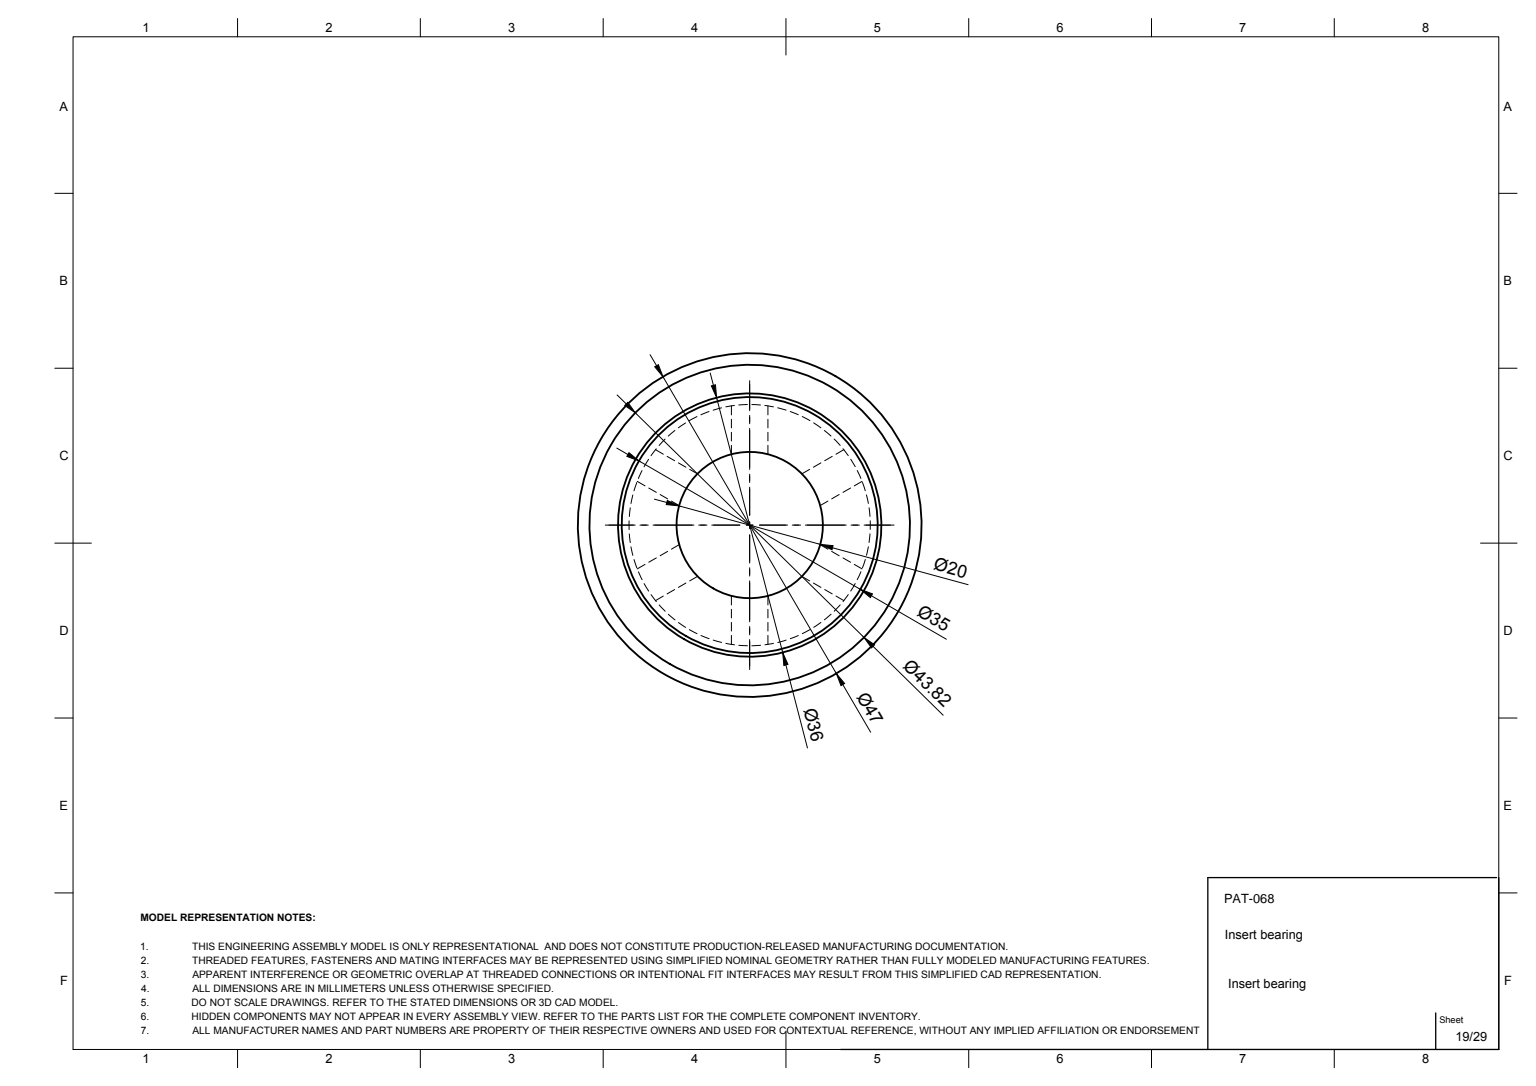
ISO-10303-21;
HEADER;
/* Generated by software containing ST-Developer
 * from STEP Tools, Inc. (www.steptools.com) 
 */

FILE_DESCRIPTION(
/* description */ ('Line shaft on three pillow blocks'),
/* implementation_level */ '2;1');

FILE_NAME(
/* name */ 'Insert bearing.step',
/* time_stamp */ '2026-10-27T10:49:19-07:00',
/* author */ (''),
/* organization */ (''),
/* preprocessor_version */ 'ST-DEVELOPER v20.2',
/* originating_system */ 'Autodesk Translation Framework v15.17.0.0',
/* authorisation */ '');

FILE_SCHEMA (('AUTOMOTIVE_DESIGN { 1 0 10303 214 3 1 1 }'));
ENDSEC;

DATA;
#10=MECHANICAL_DESIGN_GEOMETRIC_PRESENTATION_REPRESENTATION('',(#352,#353),#8377);
#223=B_SPLINE_CURVE_WITH_KNOTS('',3,(#7015,#7016,#7017,#7018,#7019,#7020,
#7021,#7022,#7023,#7024),.UNSPECIFIED.,.F.,.F.,(4,2,2,2,4),(1.13193471301885,
1.22626174930539,1.32058878559194,1.41491753480854,1.50924628402513),
 .UNSPECIFIED.);
#224=B_SPLINE_CURVE_WITH_KNOTS('',3,(#7026,#7027,#7028,#7029,#7030,#7031,
#7032,#7033,#7034,#7035,#7036,#7037,#7038,#7039,#7040,#7041,#7042,#7043),
 .UNSPECIFIED.,.F.,.F.,(4,2,2,2,2,2,2,2,4),(0.377311571006283,0.471638607292829,
0.565965643579376,0.66029439279597,0.754623142012565,0.84895189122916,0.943280640445754,
1.0376076767323,1.13193471301885),.UNSPECIFIED.);
#225=B_SPLINE_CURVE_WITH_KNOTS('',3,(#7044,#7045,#7046,#7047,#7048,#7049,
#7050,#7051,#7052,#7053),.UNSPECIFIED.,.F.,.F.,(4,2,2,2,4),(1.50924628402513,
1.60357503324173,1.69790378245832,1.79223081874487,1.88655785503141),
 .UNSPECIFIED.);
#226=B_SPLINE_CURVE_WITH_KNOTS('',3,(#7056,#7057,#7058,#7059,#7060,#7061,
#7062,#7063,#7064,#7065,#7066,#7067,#7068,#7069,#7070,#7071,#7072,#7073,
#7074,#7075,#7076,#7077,#7078,#7079,#7080,#7081,#7082,#7083,#7084,#7085,
#7086,#7087,#7088,#7089),.UNSPECIFIED.,.T.,.F.,(4,2,2,2,2,2,2,2,2,2,2,2,
2,2,2,2,4),(0.,0.0946120580087934,0.189224116017587,0.283822945575014,0.378421775132442,
0.47302060468987,0.567619434247297,0.662231492256091,0.756843550264884,
0.851455608273677,0.94606766628247,1.0406664958399,1.13526532539733,1.22986415495475,
1.32446298451218,1.41907504252097,1.51368710052977),.UNSPECIFIED.);
#227=B_SPLINE_CURVE_WITH_KNOTS('',3,(#7092,#7093,#7094,#7095,#7096,#7097,
#7098,#7099,#7100,#7101,#7102,#7103,#7104,#7105,#7106,#7107,#7108,#7109,
#7110,#7111,#7112,#7113,#7114,#7115,#7116,#7117,#7118,#7119,#7120,#7121,
#7122,#7123,#7124,#7125),.UNSPECIFIED.,.T.,.F.,(4,2,2,2,2,2,2,2,2,2,2,2,
2,2,2,2,4),(0.,0.0946120580087934,0.189224116017587,0.283822945575014,0.378421775132442,
0.47302060468987,0.567619434247297,0.66223149225609,0.756843550264884,0.851455608273677,
0.94606766628247,1.0406664958399,1.13526532539733,1.22986415495475,1.32446298451218,
1.41907504252097,1.51368710052977),.UNSPECIFIED.);
#228=B_SPLINE_CURVE_WITH_KNOTS('',3,(#7129,#7130,#7131,#7132,#7133,#7134,
#7135,#7136,#7137,#7138),.UNSPECIFIED.,.F.,.F.,(4,2,2,2,4),(1.13193471301885,
1.22626174930539,1.32058878559194,1.41491753480854,1.50924628402513),
 .UNSPECIFIED.);
#229=B_SPLINE_CURVE_WITH_KNOTS('',3,(#7140,#7141,#7142,#7143,#7144,#7145,
#7146,#7147,#7148,#7149,#7150,#7151,#7152,#7153,#7154,#7155,#7156,#7157),
 .UNSPECIFIED.,.F.,.F.,(4,2,2,2,2,2,2,2,4),(0.377311571006283,0.47163860729283,
0.565965643579376,0.660294392795971,0.754623142012565,0.84895189122916,
0.943280640445755,1.0376076767323,1.13193471301885),.UNSPECIFIED.);
#230=B_SPLINE_CURVE_WITH_KNOTS('',3,(#7158,#7159,#7160,#7161,#7162,#7163,
#7164,#7165,#7166,#7167),.UNSPECIFIED.,.F.,.F.,(4,2,2,2,4),(1.50924628402513,
1.60357503324173,1.69790378245832,1.79223081874487,1.88655785503141),
 .UNSPECIFIED.);
#231=B_SPLINE_CURVE_WITH_KNOTS('',3,(#7176,#7177,#7178,#7179,#7180,#7181,
#7182,#7183,#7184,#7185,#7186,#7187,#7188,#7189,#7190,#7191,#7192,#7193),
 .UNSPECIFIED.,.F.,.F.,(4,2,2,2,2,2,2,2,4),(0.377311571006282,0.471638607292829,
0.565965643579376,0.660294392795971,0.754623142012565,0.84895189122916,
0.943280640445754,1.0376076767323,1.13193471301885),.UNSPECIFIED.);
#232=B_SPLINE_CURVE_WITH_KNOTS('',3,(#7195,#7196,#7197,#7198,#7199,#7200,
#7201,#7202,#7203,#7204),.UNSPECIFIED.,.F.,.F.,(4,2,2,2,4),(1.13193471301885,
1.22626174930539,1.32058878559194,1.41491753480854,1.50924628402513),
 .UNSPECIFIED.);
#233=B_SPLINE_CURVE_WITH_KNOTS('',3,(#7205,#7206,#7207,#7208,#7209,#7210,
#7211,#7212,#7213,#7214),.UNSPECIFIED.,.F.,.F.,(4,2,2,2,4),(1.50924628402513,
1.60357503324172,1.69790378245832,1.79223081874487,1.88655785503141),
 .UNSPECIFIED.);
#234=B_SPLINE_CURVE_WITH_KNOTS('',3,(#7217,#7218,#7219,#7220,#7221,#7222,
#7223,#7224,#7225,#7226,#7227,#7228,#7229,#7230,#7231,#7232,#7233,#7234),
 .UNSPECIFIED.,.F.,.F.,(4,2,2,2,2,2,2,2,4),(0.377311571006283,0.47163860729283,
0.565965643579376,0.660294392795971,0.754623142012565,0.84895189122916,
0.943280640445754,1.0376076767323,1.13193471301885),.UNSPECIFIED.);
#235=B_SPLINE_CURVE_WITH_KNOTS('',3,(#7236,#7237,#7238,#7239,#7240,#7241,
#7242,#7243,#7244,#7245),.UNSPECIFIED.,.F.,.F.,(4,2,2,2,4),(1.13193471301885,
1.22626174930539,1.32058878559194,1.41491753480854,1.50924628402513),
 .UNSPECIFIED.);
#236=B_SPLINE_CURVE_WITH_KNOTS('',3,(#7246,#7247,#7248,#7249,#7250,#7251,
#7252,#7253,#7254,#7255),.UNSPECIFIED.,.F.,.F.,(4,2,2,2,4),(1.50924628402513,
1.60357503324173,1.69790378245832,1.79223081874487,1.88655785503141),
 .UNSPECIFIED.);
#237=B_SPLINE_CURVE_WITH_KNOTS('',3,(#7258,#7259,#7260,#7261,#7262,#7263,
#7264,#7265,#7266,#7267,#7268,#7269,#7270,#7271,#7272,#7273,#7274,#7275),
 .UNSPECIFIED.,.F.,.F.,(4,2,2,2,2,2,2,2,4),(0.377311571006282,0.471638607292829,
0.565965643579376,0.66029439279597,0.754623142012565,0.84895189122916,0.943280640445754,
1.0376076767323,1.13193471301885),.UNSPECIFIED.);
#238=B_SPLINE_CURVE_WITH_KNOTS('',3,(#7277,#7278,#7279,#7280,#7281,#7282,
#7283,#7284,#7285,#7286),.UNSPECIFIED.,.F.,.F.,(4,2,2,2,4),(1.13193471301885,
1.22626174930539,1.32058878559194,1.41491753480854,1.50924628402513),
 .UNSPECIFIED.);
#239=B_SPLINE_CURVE_WITH_KNOTS('',3,(#7287,#7288,#7289,#7290,#7291,#7292,
#7293,#7294,#7295,#7296),.UNSPECIFIED.,.F.,.F.,(4,2,2,2,4),(1.50924628402513,
1.60357503324172,1.69790378245832,1.79223081874487,1.88655785503141),
 .UNSPECIFIED.);
#240=B_SPLINE_CURVE_WITH_KNOTS('',3,(#7299,#7300,#7301,#7302,#7303,#7304,
#7305,#7306,#7307,#7308,#7309,#7310,#7311,#7312,#7313,#7314,#7315,#7316),
 .UNSPECIFIED.,.F.,.F.,(4,2,2,2,2,2,2,2,4),(0.377311571006283,0.471638607292829,
0.565965643579376,0.660294392795971,0.754623142012565,0.84895189122916,
0.943280640445755,1.0376076767323,1.13193471301885),.UNSPECIFIED.);
#241=B_SPLINE_CURVE_WITH_KNOTS('',3,(#7318,#7319,#7320,#7321,#7322,#7323,
#7324,#7325,#7326,#7327),.UNSPECIFIED.,.F.,.F.,(4,2,2,2,4),(1.13193471301885,
1.22626174930539,1.32058878559194,1.41491753480854,1.50924628402513),
 .UNSPECIFIED.);
#242=B_SPLINE_CURVE_WITH_KNOTS('',3,(#7328,#7329,#7330,#7331,#7332,#7333,
#7334,#7335,#7336,#7337),.UNSPECIFIED.,.F.,.F.,(4,2,2,2,4),(1.50924628402513,
1.60357503324172,1.69790378245832,1.79223081874487,1.88655785503141),
 .UNSPECIFIED.);
#243=B_SPLINE_CURVE_WITH_KNOTS('',3,(#7341,#7342,#7343,#7344,#7345,#7346,
#7347,#7348,#7349,#7350,#7351,#7352,#7353,#7354,#7355,#7356,#7357,#7358,
#7359,#7360,#7361,#7362,#7363,#7364,#7365,#7366,#7367,#7368,#7369,#7370,
#7371,#7372,#7373,#7374),.UNSPECIFIED.,.T.,.F.,(4,2,2,2,2,2,2,2,2,2,2,2,
2,2,2,2,4),(0.,0.0946120580087934,0.189224116017587,0.283822945575014,0.378421775132442,
0.47302060468987,0.567619434247297,0.66223149225609,0.756843550264884,0.851455608273677,
0.94606766628247,1.0406664958399,1.13526532539733,1.22986415495475,1.32446298451218,
1.41907504252097,1.51368710052977),.UNSPECIFIED.);
#244=B_SPLINE_CURVE_WITH_KNOTS('',3,(#7377,#7378,#7379,#7380,#7381,#7382,
#7383,#7384,#7385,#7386,#7387,#7388,#7389,#7390,#7391,#7392,#7393,#7394,
#7395,#7396,#7397,#7398,#7399,#7400,#7401,#7402,#7403,#7404,#7405,#7406,
#7407,#7408,#7409,#7410),.UNSPECIFIED.,.T.,.F.,(4,2,2,2,2,2,2,2,2,2,2,2,
2,2,2,2,4),(0.,0.0946120580087934,0.189224116017587,0.283822945575014,0.378421775132442,
0.47302060468987,0.567619434247297,0.66223149225609,0.756843550264884,0.851455608273677,
0.94606766628247,1.0406664958399,1.13526532539733,1.22986415495475,1.32446298451218,
1.41907504252097,1.51368710052977),.UNSPECIFIED.);
#245=B_SPLINE_CURVE_WITH_KNOTS('',3,(#7415,#7416,#7417,#7418,#7419,#7420,
#7421,#7422,#7423,#7424,#7425,#7426,#7427,#7428,#7429,#7430,#7431,#7432,
#7433,#7434,#7435,#7436,#7437,#7438,#7439,#7440,#7441,#7442,#7443,#7444,
#7445,#7446,#7447,#7448),.UNSPECIFIED.,.T.,.F.,(4,2,2,2,2,2,2,2,2,2,2,2,
2,2,2,2,4),(0.,0.0946120580087934,0.189224116017587,0.283822945575014,0.378421775132442,
0.47302060468987,0.567619434247297,0.66223149225609,0.756843550264884,0.851455608273677,
0.94606766628247,1.0406664958399,1.13526532539733,1.22986415495475,1.32446298451218,
1.41907504252097,1.51368710052977),.UNSPECIFIED.);
#246=B_SPLINE_CURVE_WITH_KNOTS('',3,(#7451,#7452,#7453,#7454,#7455,#7456,
#7457,#7458,#7459,#7460,#7461,#7462,#7463,#7464,#7465,#7466,#7467,#7468,
#7469,#7470,#7471,#7472,#7473,#7474,#7475,#7476,#7477,#7478,#7479,#7480,
#7481,#7482,#7483,#7484),.UNSPECIFIED.,.T.,.F.,(4,2,2,2,2,2,2,2,2,2,2,2,
2,2,2,2,4),(0.,0.0946120580087934,0.189224116017587,0.283822945575014,0.378421775132442,
0.47302060468987,0.567619434247297,0.66223149225609,0.756843550264884,0.851455608273677,
0.94606766628247,1.0406664958399,1.13526532539733,1.22986415495475,1.32446298451218,
1.41907504252097,1.51368710052977),.UNSPECIFIED.);
#264=SPHERICAL_SURFACE('',#4873,2.35);
#298=SHAPE_REPRESENTATION_RELATIONSHIP('SRR','None',#8514,#325);
#325=ADVANCED_BREP_SHAPE_REPRESENTATION('',(#379,#380),#8363);
#352=STYLED_ITEM('',(#8718),#379);
#353=STYLED_ITEM('',(#8718),#380);
#379=MANIFOLD_SOLID_BREP('Body1',#4339);
#380=MANIFOLD_SOLID_BREP('Body2',#4340);
#440=FACE_BOUND('',#1075,.T.);
#441=FACE_BOUND('',#1077,.T.);
#442=FACE_BOUND('',#1078,.T.);
#443=FACE_BOUND('',#1080,.T.);
#444=FACE_BOUND('',#1084,.T.);
#445=FACE_BOUND('',#1085,.T.);
#446=FACE_BOUND('',#1086,.T.);
#447=FACE_BOUND('',#1087,.T.);
#448=FACE_BOUND('',#1088,.T.);
#449=FACE_BOUND('',#1089,.T.);
#450=FACE_BOUND('',#1095,.T.);
#451=FACE_BOUND('',#1097,.T.);
#452=FACE_BOUND('',#1100,.T.);
#453=FACE_BOUND('',#1102,.T.);
#454=FACE_BOUND('',#1103,.T.);
#455=FACE_BOUND('',#1104,.T.);
#456=FACE_BOUND('',#1105,.T.);
#457=FACE_BOUND('',#1106,.T.);
#458=FACE_BOUND('',#1107,.T.);
#566=PLANE('',#4871);
#567=PLANE('',#4876);
#568=PLANE('',#4886);
#569=PLANE('',#4888);
#570=PLANE('',#4892);
#772=FACE_OUTER_BOUND('',#1073,.T.);
#773=FACE_OUTER_BOUND('',#1074,.T.);
#774=FACE_OUTER_BOUND('',#1076,.T.);
#775=FACE_OUTER_BOUND('',#1079,.T.);
#776=FACE_OUTER_BOUND('',#1081,.T.);
#777=FACE_OUTER_BOUND('',#1082,.T.);
#778=FACE_OUTER_BOUND('',#1083,.T.);
#779=FACE_OUTER_BOUND('',#1090,.T.);
#780=FACE_OUTER_BOUND('',#1091,.T.);
#781=FACE_OUTER_BOUND('',#1092,.T.);
#782=FACE_OUTER_BOUND('',#1093,.T.);
#783=FACE_OUTER_BOUND('',#1094,.T.);
#784=FACE_OUTER_BOUND('',#1096,.T.);
#785=FACE_OUTER_BOUND('',#1098,.T.);
#786=FACE_OUTER_BOUND('',#1099,.T.);
#787=FACE_OUTER_BOUND('',#1101,.T.);
#1073=EDGE_LOOP('',(#3423,#3424,#3425,#3426));
#1074=EDGE_LOOP('',(#3427));
#1075=EDGE_LOOP('',(#3428));
#1076=EDGE_LOOP('',(#3429,#3430));
#1077=EDGE_LOOP('',(#3431));
#1078=EDGE_LOOP('',(#3432));
#1079=EDGE_LOOP('',(#3433));
#1080=EDGE_LOOP('',(#3434));
#1081=EDGE_LOOP('',(#3435,#3436,#3437,#3438,#3439,#3440));
#1082=EDGE_LOOP('',(#3441,#3442,#3443,#3444,#3445,#3446));
#1083=EDGE_LOOP('',(#3447,#3448,#3449,#3450));
#1084=EDGE_LOOP('',(#3451,#3452,#3453));
#1085=EDGE_LOOP('',(#3454,#3455,#3456));
#1086=EDGE_LOOP('',(#3457,#3458,#3459));
#1087=EDGE_LOOP('',(#3460,#3461,#3462));
#1088=EDGE_LOOP('',(#3463,#3464,#3465));
#1089=EDGE_LOOP('',(#3466,#3467,#3468));
#1090=EDGE_LOOP('',(#3469,#3470,#3471,#3472,#3473,#3474));
#1091=EDGE_LOOP('',(#3475,#3476,#3477,#3478,#3479,#3480));
#1092=EDGE_LOOP('',(#3481,#3482,#3483,#3484,#3485,#3486));
#1093=EDGE_LOOP('',(#3487,#3488,#3489,#3490,#3491,#3492));
#1094=EDGE_LOOP('',(#3493));
#1095=EDGE_LOOP('',(#3494));
#1096=EDGE_LOOP('',(#3495));
#1097=EDGE_LOOP('',(#3496));
#1098=EDGE_LOOP('',(#3497,#3498,#3499,#3500));
#1099=EDGE_LOOP('',(#3501));
#1100=EDGE_LOOP('',(#3502));
#1101=EDGE_LOOP('',(#3503,#3504,#3505,#3506));
#1102=EDGE_LOOP('',(#3507));
#1103=EDGE_LOOP('',(#3508));
#1104=EDGE_LOOP('',(#3509));
#1105=EDGE_LOOP('',(#3510));
#1106=EDGE_LOOP('',(#3511));
#1107=EDGE_LOOP('',(#3512));
#1413=LINE('',#7000,#1740);
#1414=LINE('',#7055,#1741);
#1415=LINE('',#7127,#1742);
#1416=LINE('',#7172,#1743);
#1417=LINE('',#7340,#1744);
#1418=LINE('',#7411,#1745);
#1419=LINE('',#7414,#1746);
#1420=LINE('',#7485,#1747);
#1421=LINE('',#7495,#1748);
#1422=LINE('',#7500,#1749);
#1740=VECTOR('',#5740,1.8);
#1741=VECTOR('',#5757,0.25);
#1742=VECTOR('',#5760,0.25);
#1743=VECTOR('',#5765,1.65);
#1744=VECTOR('',#5770,0.25);
#1745=VECTOR('',#5773,0.25);
#1746=VECTOR('',#5776,0.25);
#1747=VECTOR('',#5779,0.25);
#1748=VECTOR('',#5792,1.75);
#1749=VECTOR('',#5799,1.);
#1988=CIRCLE('',#4869,1.8);
#1989=CIRCLE('',#4870,1.8);
#1990=CIRCLE('',#4872,2.19089023002066);
#1991=CIRCLE('',#4874,2.35);
#1992=CIRCLE('',#4875,2.19089023002066);
#1993=CIRCLE('',#4880,1.65);
#1994=CIRCLE('',#4881,1.65);
#1995=CIRCLE('',#4887,1.);
#1996=CIRCLE('',#4889,1.75);
#1997=CIRCLE('',#4891,1.75);
#1998=CIRCLE('',#4893,1.);
#2226=VERTEX_POINT('',#6997);
#2227=VERTEX_POINT('',#6999);
#2228=VERTEX_POINT('',#7003);
#2229=VERTEX_POINT('',#7006);
#2230=VERTEX_POINT('',#7007);
#2231=VERTEX_POINT('',#7009);
#2232=VERTEX_POINT('',#7013);
#2233=VERTEX_POINT('',#7014);
#2234=VERTEX_POINT('',#7025);
#2235=VERTEX_POINT('',#7054);
#2236=VERTEX_POINT('',#7091);
#2237=VERTEX_POINT('',#7126);
#2238=VERTEX_POINT('',#7128);
#2239=VERTEX_POINT('',#7139);
#2240=VERTEX_POINT('',#7169);
#2241=VERTEX_POINT('',#7171);
#2242=VERTEX_POINT('',#7174);
#2243=VERTEX_POINT('',#7175);
#2244=VERTEX_POINT('',#7194);
#2245=VERTEX_POINT('',#7215);
#2246=VERTEX_POINT('',#7216);
#2247=VERTEX_POINT('',#7235);
#2248=VERTEX_POINT('',#7256);
#2249=VERTEX_POINT('',#7257);
#2250=VERTEX_POINT('',#7276);
#2251=VERTEX_POINT('',#7297);
#2252=VERTEX_POINT('',#7298);
#2253=VERTEX_POINT('',#7317);
#2254=VERTEX_POINT('',#7339);
#2255=VERTEX_POINT('',#7376);
#2256=VERTEX_POINT('',#7413);
#2257=VERTEX_POINT('',#7450);
#2258=VERTEX_POINT('',#7487);
#2259=VERTEX_POINT('',#7490);
#2260=VERTEX_POINT('',#7493);
#2261=VERTEX_POINT('',#7497);
#2660=EDGE_CURVE('',#2226,#2226,#1988,.T.);
#2661=EDGE_CURVE('',#2226,#2227,#1413,.T.);
#2662=EDGE_CURVE('',#2227,#2227,#1989,.T.);
#2663=EDGE_CURVE('',#2228,#2228,#1990,.T.);
#2664=EDGE_CURVE('',#2229,#2230,#1991,.T.);
#2665=EDGE_CURVE('',#2231,#2231,#1992,.T.);
#2666=EDGE_CURVE('',#2232,#2233,#223,.T.);
#2667=EDGE_CURVE('',#2234,#2232,#224,.T.);
#2668=EDGE_CURVE('',#2233,#2234,#225,.T.);
#2669=EDGE_CURVE('',#2233,#2235,#1414,.T.);
#2670=EDGE_CURVE('',#2235,#2235,#226,.T.);
#2671=EDGE_CURVE('',#2236,#2236,#227,.T.);
#2672=EDGE_CURVE('',#2236,#2237,#1415,.T.);
#2673=EDGE_CURVE('',#2238,#2237,#228,.T.);
#2674=EDGE_CURVE('',#2239,#2238,#229,.T.);
#2675=EDGE_CURVE('',#2237,#2239,#230,.T.);
#2676=EDGE_CURVE('',#2240,#2240,#1993,.T.);
#2677=EDGE_CURVE('',#2240,#2241,#1416,.T.);
#2678=EDGE_CURVE('',#2241,#2241,#1994,.T.);
#2679=EDGE_CURVE('',#2242,#2243,#231,.T.);
#2680=EDGE_CURVE('',#2243,#2244,#232,.T.);
#2681=EDGE_CURVE('',#2244,#2242,#233,.T.);
#2682=EDGE_CURVE('',#2245,#2246,#234,.T.);
#2683=EDGE_CURVE('',#2246,#2247,#235,.T.);
#2684=EDGE_CURVE('',#2247,#2245,#236,.T.);
#2685=EDGE_CURVE('',#2248,#2249,#237,.T.);
#2686=EDGE_CURVE('',#2249,#2250,#238,.T.);
#2687=EDGE_CURVE('',#2250,#2248,#239,.T.);
#2688=EDGE_CURVE('',#2251,#2252,#240,.T.);
#2689=EDGE_CURVE('',#2252,#2253,#241,.T.);
#2690=EDGE_CURVE('',#2253,#2251,#242,.T.);
#2691=EDGE_CURVE('',#2244,#2254,#1417,.T.);
#2692=EDGE_CURVE('',#2254,#2254,#243,.T.);
#2693=EDGE_CURVE('',#2255,#2255,#244,.T.);
#2694=EDGE_CURVE('',#2255,#2247,#1418,.T.);
#2695=EDGE_CURVE('',#2250,#2256,#1419,.T.);
#2696=EDGE_CURVE('',#2256,#2256,#245,.T.);
#2697=EDGE_CURVE('',#2257,#2257,#246,.T.);
#2698=EDGE_CURVE('',#2257,#2253,#1420,.T.);
#2699=EDGE_CURVE('',#2258,#2258,#1995,.T.);
#2700=EDGE_CURVE('',#2259,#2259,#1996,.T.);
#2701=EDGE_CURVE('',#2260,#2260,#1997,.T.);
#2702=EDGE_CURVE('',#2260,#2259,#1421,.T.);
#2703=EDGE_CURVE('',#2261,#2261,#1998,.T.);
#2704=EDGE_CURVE('',#2261,#2258,#1422,.T.);
#3423=ORIENTED_EDGE('',*,*,#2660,.T.);
#3424=ORIENTED_EDGE('',*,*,#2661,.T.);
#3425=ORIENTED_EDGE('',*,*,#2662,.F.);
#3426=ORIENTED_EDGE('',*,*,#2661,.F.);
#3427=ORIENTED_EDGE('',*,*,#2663,.F.);
#3428=ORIENTED_EDGE('',*,*,#2662,.T.);
#3429=ORIENTED_EDGE('',*,*,#2664,.T.);
#3430=ORIENTED_EDGE('',*,*,#2664,.F.);
#3431=ORIENTED_EDGE('',*,*,#2663,.T.);
#3432=ORIENTED_EDGE('',*,*,#2665,.F.);
#3433=ORIENTED_EDGE('',*,*,#2665,.T.);
#3434=ORIENTED_EDGE('',*,*,#2660,.F.);
#3435=ORIENTED_EDGE('',*,*,#2666,.F.);
#3436=ORIENTED_EDGE('',*,*,#2667,.F.);
#3437=ORIENTED_EDGE('',*,*,#2668,.F.);
#3438=ORIENTED_EDGE('',*,*,#2669,.T.);
#3439=ORIENTED_EDGE('',*,*,#2670,.F.);
#3440=ORIENTED_EDGE('',*,*,#2669,.F.);
#3441=ORIENTED_EDGE('',*,*,#2671,.F.);
#3442=ORIENTED_EDGE('',*,*,#2672,.T.);
#3443=ORIENTED_EDGE('',*,*,#2673,.F.);
#3444=ORIENTED_EDGE('',*,*,#2674,.F.);
#3445=ORIENTED_EDGE('',*,*,#2675,.F.);
#3446=ORIENTED_EDGE('',*,*,#2672,.F.);
#3447=ORIENTED_EDGE('',*,*,#2676,.F.);
#3448=ORIENTED_EDGE('',*,*,#2677,.T.);
#3449=ORIENTED_EDGE('',*,*,#2678,.T.);
#3450=ORIENTED_EDGE('',*,*,#2677,.F.);
#3451=ORIENTED_EDGE('',*,*,#2667,.T.);
#3452=ORIENTED_EDGE('',*,*,#2666,.T.);
#3453=ORIENTED_EDGE('',*,*,#2668,.T.);
#3454=ORIENTED_EDGE('',*,*,#2674,.T.);
#3455=ORIENTED_EDGE('',*,*,#2673,.T.);
#3456=ORIENTED_EDGE('',*,*,#2675,.T.);
#3457=ORIENTED_EDGE('',*,*,#2679,.T.);
#3458=ORIENTED_EDGE('',*,*,#2680,.T.);
#3459=ORIENTED_EDGE('',*,*,#2681,.T.);
#3460=ORIENTED_EDGE('',*,*,#2682,.T.);
#3461=ORIENTED_EDGE('',*,*,#2683,.T.);
#3462=ORIENTED_EDGE('',*,*,#2684,.T.);
#3463=ORIENTED_EDGE('',*,*,#2685,.T.);
#3464=ORIENTED_EDGE('',*,*,#2686,.T.);
#3465=ORIENTED_EDGE('',*,*,#2687,.T.);
#3466=ORIENTED_EDGE('',*,*,#2688,.T.);
#3467=ORIENTED_EDGE('',*,*,#2689,.T.);
#3468=ORIENTED_EDGE('',*,*,#2690,.T.);
#3469=ORIENTED_EDGE('',*,*,#2680,.F.);
#3470=ORIENTED_EDGE('',*,*,#2679,.F.);
#3471=ORIENTED_EDGE('',*,*,#2681,.F.);
#3472=ORIENTED_EDGE('',*,*,#2691,.T.);
#3473=ORIENTED_EDGE('',*,*,#2692,.F.);
#3474=ORIENTED_EDGE('',*,*,#2691,.F.);
#3475=ORIENTED_EDGE('',*,*,#2693,.F.);
#3476=ORIENTED_EDGE('',*,*,#2694,.T.);
#3477=ORIENTED_EDGE('',*,*,#2683,.F.);
#3478=ORIENTED_EDGE('',*,*,#2682,.F.);
#3479=ORIENTED_EDGE('',*,*,#2684,.F.);
#3480=ORIENTED_EDGE('',*,*,#2694,.F.);
#3481=ORIENTED_EDGE('',*,*,#2686,.F.);
#3482=ORIENTED_EDGE('',*,*,#2685,.F.);
#3483=ORIENTED_EDGE('',*,*,#2687,.F.);
#3484=ORIENTED_EDGE('',*,*,#2695,.T.);
#3485=ORIENTED_EDGE('',*,*,#2696,.F.);
#3486=ORIENTED_EDGE('',*,*,#2695,.F.);
#3487=ORIENTED_EDGE('',*,*,#2697,.F.);
#3488=ORIENTED_EDGE('',*,*,#2698,.T.);
#3489=ORIENTED_EDGE('',*,*,#2689,.F.);
#3490=ORIENTED_EDGE('',*,*,#2688,.F.);
#3491=ORIENTED_EDGE('',*,*,#2690,.F.);
#3492=ORIENTED_EDGE('',*,*,#2698,.F.);
#3493=ORIENTED_EDGE('',*,*,#2678,.F.);
#3494=ORIENTED_EDGE('',*,*,#2699,.T.);
#3495=ORIENTED_EDGE('',*,*,#2700,.F.);
#3496=ORIENTED_EDGE('',*,*,#2676,.T.);
#3497=ORIENTED_EDGE('',*,*,#2701,.F.);
#3498=ORIENTED_EDGE('',*,*,#2702,.T.);
#3499=ORIENTED_EDGE('',*,*,#2700,.T.);
#3500=ORIENTED_EDGE('',*,*,#2702,.F.);
#3501=ORIENTED_EDGE('',*,*,#2701,.T.);
#3502=ORIENTED_EDGE('',*,*,#2703,.F.);
#3503=ORIENTED_EDGE('',*,*,#2703,.T.);
#3504=ORIENTED_EDGE('',*,*,#2704,.T.);
#3505=ORIENTED_EDGE('',*,*,#2699,.F.);
#3506=ORIENTED_EDGE('',*,*,#2704,.F.);
#3507=ORIENTED_EDGE('',*,*,#2671,.T.);
#3508=ORIENTED_EDGE('',*,*,#2670,.T.);
#3509=ORIENTED_EDGE('',*,*,#2693,.T.);
#3510=ORIENTED_EDGE('',*,*,#2692,.T.);
#3511=ORIENTED_EDGE('',*,*,#2697,.T.);
#3512=ORIENTED_EDGE('',*,*,#2696,.T.);
#4036=CYLINDRICAL_SURFACE('',#4868,1.8);
#4037=CYLINDRICAL_SURFACE('',#4877,0.25);
#4038=CYLINDRICAL_SURFACE('',#4878,0.25);
#4039=CYLINDRICAL_SURFACE('',#4879,1.65);
#4040=CYLINDRICAL_SURFACE('',#4882,0.25);
#4041=CYLINDRICAL_SURFACE('',#4883,0.25);
#4042=CYLINDRICAL_SURFACE('',#4884,0.25);
#4043=CYLINDRICAL_SURFACE('',#4885,0.25);
#4044=CYLINDRICAL_SURFACE('',#4890,1.75);
#4045=CYLINDRICAL_SURFACE('',#4894,1.);
#4190=ADVANCED_FACE('',(#772),#4036,.F.);
#4191=ADVANCED_FACE('',(#773,#440),#566,.T.);
#4192=ADVANCED_FACE('',(#774,#441,#442),#264,.T.);
#4193=ADVANCED_FACE('',(#775,#443),#567,.T.);
#4194=ADVANCED_FACE('',(#776),#4037,.F.);
#4195=ADVANCED_FACE('',(#777),#4038,.F.);
#4196=ADVANCED_FACE('',(#778,#444,#445,#446,#447,#448,#449),#4039,.T.);
#4197=ADVANCED_FACE('',(#779),#4040,.F.);
#4198=ADVANCED_FACE('',(#780),#4041,.F.);
#4199=ADVANCED_FACE('',(#781),#4042,.F.);
#4200=ADVANCED_FACE('',(#782),#4043,.F.);
#4201=ADVANCED_FACE('',(#783,#450),#568,.T.);
#4202=ADVANCED_FACE('',(#784,#451),#569,.T.);
#4203=ADVANCED_FACE('',(#785),#4044,.T.);
#4204=ADVANCED_FACE('',(#786,#452),#570,.T.);
#4205=ADVANCED_FACE('',(#787,#453,#454,#455,#456,#457,#458),#4045,.F.);
#4339=CLOSED_SHELL('',(#4190,#4191,#4192,#4193));
#4340=CLOSED_SHELL('',(#4194,#4195,#4196,#4197,#4198,#4199,#4200,#4201,
#4202,#4203,#4204,#4205));
#4867=AXIS2_PLACEMENT_3D('',#6995,#5734,#5735);
#4868=AXIS2_PLACEMENT_3D('',#6996,#5736,#5737);
#4869=AXIS2_PLACEMENT_3D('',#6998,#5738,#5739);
#4870=AXIS2_PLACEMENT_3D('',#7001,#5741,#5742);
#4871=AXIS2_PLACEMENT_3D('',#7002,#5743,#5744);
#4872=AXIS2_PLACEMENT_3D('',#7004,#5745,#5746);
#4873=AXIS2_PLACEMENT_3D('',#7005,#5747,#5748);
#4874=AXIS2_PLACEMENT_3D('',#7008,#5749,#5750);
#4875=AXIS2_PLACEMENT_3D('',#7010,#5751,#5752);
#4876=AXIS2_PLACEMENT_3D('',#7011,#5753,#5754);
#4877=AXIS2_PLACEMENT_3D('',#7012,#5755,#5756);
#4878=AXIS2_PLACEMENT_3D('',#7090,#5758,#5759);
#4879=AXIS2_PLACEMENT_3D('',#7168,#5761,#5762);
#4880=AXIS2_PLACEMENT_3D('',#7170,#5763,#5764);
#4881=AXIS2_PLACEMENT_3D('',#7173,#5766,#5767);
#4882=AXIS2_PLACEMENT_3D('',#7338,#5768,#5769);
#4883=AXIS2_PLACEMENT_3D('',#7375,#5771,#5772);
#4884=AXIS2_PLACEMENT_3D('',#7412,#5774,#5775);
#4885=AXIS2_PLACEMENT_3D('',#7449,#5777,#5778);
#4886=AXIS2_PLACEMENT_3D('',#7486,#5780,#5781);
#4887=AXIS2_PLACEMENT_3D('',#7488,#5782,#5783);
#4888=AXIS2_PLACEMENT_3D('',#7489,#5784,#5785);
#4889=AXIS2_PLACEMENT_3D('',#7491,#5786,#5787);
#4890=AXIS2_PLACEMENT_3D('',#7492,#5788,#5789);
#4891=AXIS2_PLACEMENT_3D('',#7494,#5790,#5791);
#4892=AXIS2_PLACEMENT_3D('',#7496,#5793,#5794);
#4893=AXIS2_PLACEMENT_3D('',#7498,#5795,#5796);
#4894=AXIS2_PLACEMENT_3D('',#7499,#5797,#5798);
#5734=DIRECTION('axis',(0.,0.,1.));
#5735=DIRECTION('refdir',(1.,0.,0.));
#5736=DIRECTION('center_axis',(0.,-1.,0.));
#5737=DIRECTION('ref_axis',(1.,0.,0.));
#5738=DIRECTION('center_axis',(0.,-1.,0.));
#5739=DIRECTION('ref_axis',(1.,0.,0.));
#5740=DIRECTION('',(0.,1.,0.));
#5741=DIRECTION('center_axis',(0.,-1.,0.));
#5742=DIRECTION('ref_axis',(1.,0.,0.));
#5743=DIRECTION('center_axis',(0.,1.,0.));
#5744=DIRECTION('ref_axis',(0.,0.,1.));
#5745=DIRECTION('center_axis',(0.,-1.,0.));
#5746=DIRECTION('ref_axis',(1.,0.,0.));
#5747=DIRECTION('center_axis',(6.12323399573677E-17,0.,1.));
#5748=DIRECTION('ref_axis',(1.,0.,0.));
#5749=DIRECTION('center_axis',(1.22464679914735E-16,-1.,0.));
#5750=DIRECTION('ref_axis',(-1.,-1.22464679914735E-16,0.));
#5751=DIRECTION('center_axis',(0.,-1.,0.));
#5752=DIRECTION('ref_axis',(1.,0.,0.));
#5753=DIRECTION('center_axis',(0.,-1.,0.));
#5754=DIRECTION('ref_axis',(0.,0.,-1.));
#5755=DIRECTION('center_axis',(-0.866025403784438,0.,-0.5));
#5756=DIRECTION('ref_axis',(-0.5,0.,0.866025403784438));
#5757=DIRECTION('',(-0.866025403784438,0.,-0.5));
#5758=DIRECTION('center_axis',(-0.866025403784438,0.,-0.5));
#5759=DIRECTION('ref_axis',(-0.5,0.,0.866025403784438));
#5760=DIRECTION('',(-0.866025403784438,0.,-0.5));
#5761=DIRECTION('center_axis',(0.,-1.,0.));
#5762=DIRECTION('ref_axis',(1.,0.,0.));
#5763=DIRECTION('center_axis',(0.,-1.,0.));
#5764=DIRECTION('ref_axis',(1.,0.,0.));
#5765=DIRECTION('',(0.,1.,0.));
#5766=DIRECTION('center_axis',(0.,-1.,0.));
#5767=DIRECTION('ref_axis',(1.,0.,0.));
#5768=DIRECTION('center_axis',(0.866025403784439,0.,-0.5));
#5769=DIRECTION('ref_axis',(-0.5,0.,-0.866025403784439));
#5770=DIRECTION('',(0.866025403784439,0.,-0.5));
#5771=DIRECTION('center_axis',(0.866025403784439,0.,-0.5));
#5772=DIRECTION('ref_axis',(-0.5,0.,-0.866025403784439));
#5773=DIRECTION('',(0.866025403784439,0.,-0.5));
#5774=DIRECTION('center_axis',(0.,0.,1.));
#5775=DIRECTION('ref_axis',(1.,0.,0.));
#5776=DIRECTION('',(0.,0.,1.));
#5777=DIRECTION('center_axis',(0.,0.,1.));
#5778=DIRECTION('ref_axis',(1.,0.,0.));
#5779=DIRECTION('',(0.,0.,1.));
#5780=DIRECTION('center_axis',(0.,1.,0.));
#5781=DIRECTION('ref_axis',(0.,0.,1.));
#5782=DIRECTION('center_axis',(0.,-1.,0.));
#5783=DIRECTION('ref_axis',(1.,0.,0.));
#5784=DIRECTION('center_axis',(0.,1.,0.));
#5785=DIRECTION('ref_axis',(0.,0.,1.));
#5786=DIRECTION('center_axis',(0.,-1.,0.));
#5787=DIRECTION('ref_axis',(1.,0.,0.));
#5788=DIRECTION('center_axis',(0.,-1.,0.));
#5789=DIRECTION('ref_axis',(1.,0.,0.));
#5790=DIRECTION('center_axis',(0.,-1.,0.));
#5791=DIRECTION('ref_axis',(1.,0.,0.));
#5792=DIRECTION('',(0.,1.,0.));
#5793=DIRECTION('center_axis',(0.,-1.,0.));
#5794=DIRECTION('ref_axis',(0.,0.,-1.));
#5795=DIRECTION('center_axis',(0.,-1.,0.));
#5796=DIRECTION('ref_axis',(1.,0.,0.));
#5797=DIRECTION('center_axis',(0.,-1.,0.));
#5798=DIRECTION('ref_axis',(1.,0.,0.));
#5799=DIRECTION('',(0.,1.,0.));
#6995=CARTESIAN_POINT('',(0.,0.,0.));
#6996=CARTESIAN_POINT('Origin',(0.,0.,0.));
#6997=CARTESIAN_POINT('',(-1.8,-0.85,-2.20436423846524E-16));
#6998=CARTESIAN_POINT('Origin',(0.,-0.85,0.));
#6999=CARTESIAN_POINT('',(-1.8,0.85,-2.20436423846524E-16));
#7000=CARTESIAN_POINT('',(-1.8,0.,-2.20436423846524E-16));
#7001=CARTESIAN_POINT('Origin',(0.,0.85,0.));
#7002=CARTESIAN_POINT('Origin',(2.19089023002066,0.85,0.));
#7003=CARTESIAN_POINT('',(2.19089023002066,0.85,0.));
#7004=CARTESIAN_POINT('Origin',(0.,0.85,0.));
#7005=CARTESIAN_POINT('Origin',(3.99680288865056E-15,0.,0.));
#7006=CARTESIAN_POINT('',(3.85290688975075E-15,-1.76221774462768E-32,2.35));
#7007=CARTESIAN_POINT('',(3.85290688975075E-15,-1.76221774462768E-32,-2.35));
#7008=CARTESIAN_POINT('Origin',(3.99680288865056E-15,0.,0.));
#7009=CARTESIAN_POINT('',(2.19089023002066,-0.85,0.));
#7010=CARTESIAN_POINT('Origin',(0.,-0.85,0.));
#7011=CARTESIAN_POINT('Origin',(1.8,-0.85,0.));
#7012=CARTESIAN_POINT('Origin',(0.,1.55,0.));
#7013=CARTESIAN_POINT('',(1.42894191624432,1.8,0.825000000000001));
#7014=CARTESIAN_POINT('',(1.53744468918255,1.55,0.598968970568896));
#7015=CARTESIAN_POINT('Ctrl Pts',(1.42894191624432,1.8,0.825000000000001));
#7016=CARTESIAN_POINT('Ctrl Pts',(1.44466308895875,1.8,0.797770130104052));
#7017=CARTESIAN_POINT('Ctrl Pts',(1.46055812562105,1.79370633789704,0.768258557763732));
#7018=CARTESIAN_POINT('Ctrl Pts',(1.48824888379079,1.76817777258318,0.713138492740816));
#7019=CARTESIAN_POINT('Ctrl Pts',(1.50008999307766,1.74894552961493,0.687551581002689));
#7020=CARTESIAN_POINT('Ctrl Pts',(1.51812136280714,1.70460745840382,0.646764802471699));
#7021=CARTESIAN_POINT('Ctrl Pts',(1.52552758004446,1.67652816181843,0.628833667319578));
#7022=CARTESIAN_POINT('Ctrl Pts',(1.53516661651472,1.61494799959182,0.604921184808251));
#7023=CARTESIAN_POINT('Ctrl Pts',(1.53744468918255,1.58144291640553,0.598968970568896));
#7024=CARTESIAN_POINT('Ctrl Pts',(1.53744468918255,1.55,0.598968970568896));
#7025=CARTESIAN_POINT('',(1.42894191624432,1.3,0.825000000000001));
#7026=CARTESIAN_POINT('Ctrl Pts',(1.42894191624432,1.3,0.825000000000001));
#7027=CARTESIAN_POINT('Ctrl Pts',(1.4132207435299,1.3,0.852229869895949));
#7028=CARTESIAN_POINT('Ctrl Pts',(1.39561049050871,1.30629366210296,0.880751161609749));
#7029=CARTESIAN_POINT('Ctrl Pts',(1.36172049302549,1.33182222741682,0.932292094146256));
#7030=CARTESIAN_POINT('Ctrl Pts',(1.34548213209931,1.35105447038507,0.955340251466734));
#7031=CARTESIAN_POINT('Ctrl Pts',(1.31917543061769,1.39539254159618,0.99134926498299));
#7032=CARTESIAN_POINT('Ctrl Pts',(1.30734972067592,1.42347183818157,1.00672880483252));
#7033=CARTESIAN_POINT('Ctrl Pts',(1.29146042158868,1.48505200040818,1.02703269653942));
#7034=CARTESIAN_POINT('Ctrl Pts',(1.28744468918255,1.51855708359447,1.03198167246111));
#7035=CARTESIAN_POINT('Ctrl Pts',(1.28744468918255,1.58144291640553,1.03198167246111));
#7036=CARTESIAN_POINT('Ctrl Pts',(1.29146042158868,1.61494799959182,1.02703269653942));
#7037=CARTESIAN_POINT('Ctrl Pts',(1.30734972067592,1.67652816181843,1.00672880483252));
#7038=CARTESIAN_POINT('Ctrl Pts',(1.31917543061769,1.70460745840382,0.991349264982991));
#7039=CARTESIAN_POINT('Ctrl Pts',(1.34548213209931,1.74894552961493,0.955340251466735));
#7040=CARTESIAN_POINT('Ctrl Pts',(1.36172049302549,1.76817777258318,0.932292094146256));
#7041=CARTESIAN_POINT('Ctrl Pts',(1.39561049050871,1.79370633789704,0.880751161609749));
#7042=CARTESIAN_POINT('Ctrl Pts',(1.4132207435299,1.8,0.85222986989595));
#7043=CARTESIAN_POINT('Ctrl Pts',(1.42894191624432,1.8,0.825000000000001));
#7044=CARTESIAN_POINT('Ctrl Pts',(1.53744468918255,1.55,0.598968970568896));
#7045=CARTESIAN_POINT('Ctrl Pts',(1.53744468918255,1.51855708359447,0.598968970568896));
#7046=CARTESIAN_POINT('Ctrl Pts',(1.53516661651472,1.48505200040818,0.60492118480825));
#7047=CARTESIAN_POINT('Ctrl Pts',(1.52552758004446,1.42347183818157,0.628833667319578));
#7048=CARTESIAN_POINT('Ctrl Pts',(1.51812136280714,1.39539254159618,0.646764802471699));
#7049=CARTESIAN_POINT('Ctrl Pts',(1.50008999307766,1.35105447038507,0.687551581002689));
#7050=CARTESIAN_POINT('Ctrl Pts',(1.48824888379079,1.33182222741682,0.713138492740816));
#7051=CARTESIAN_POINT('Ctrl Pts',(1.46055812562105,1.30629366210296,0.768258557763732));
#7052=CARTESIAN_POINT('Ctrl Pts',(1.44466308895875,1.3,0.797770130104052));
#7053=CARTESIAN_POINT('Ctrl Pts',(1.42894191624432,1.3,0.825000000000001));
#7054=CARTESIAN_POINT('',(0.963525491562421,1.55,0.267616567329818));
#7055=CARTESIAN_POINT('',(0.125,1.55,-0.21650635094611));
#7056=CARTESIAN_POINT('Ctrl Pts',(0.963525491562421,1.55,0.267616567329818));
#7057=CARTESIAN_POINT('Ctrl Pts',(0.963525491562421,1.5815373526696,0.267616567329818));
#7058=CARTESIAN_POINT('Ctrl Pts',(0.961833761492987,1.61508042700263,0.273949373987484));
#7059=CARTESIAN_POINT('Ctrl Pts',(0.954308486908894,1.67663267125761,0.299111603474268));
#7060=CARTESIAN_POINT('Ctrl Pts',(0.948394987258249,1.70465411363682,0.31788699900678));
#7061=CARTESIAN_POINT('Ctrl Pts',(0.933155485613026,1.74889618382539,0.360174810895352));
#7062=CARTESIAN_POINT('Ctrl Pts',(0.92278792026947,1.76811531482682,0.386546956384144));
#7063=CARTESIAN_POINT('Ctrl Pts',(0.897143218189782,1.79367084275751,0.442820664919227));
#7064=CARTESIAN_POINT('Ctrl Pts',(0.881791875377343,1.8,0.472691670144998));
#7065=CARTESIAN_POINT('Ctrl Pts',(0.850258932191534,1.8,0.527308329855003));
#7066=CARTESIAN_POINT('Ctrl Pts',(0.832065554235658,1.79367084275751,0.555538485325664));
#7067=CARTESIAN_POINT('Ctrl Pts',(0.796153444118959,1.76811531482682,0.605884303066698));
#7068=CARTESIAN_POINT('Ctrl Pts',(0.778498278845144,1.74889618382539,0.62804895077401));
#7069=CARTESIAN_POINT('Ctrl Pts',(0.749495710301794,1.70465411363682,0.662390652284073));
#7070=CARTESIAN_POINT('Ctrl Pts',(0.73619249062986,1.67663267125761,0.676899590973058));
#7071=CARTESIAN_POINT('Ctrl Pts',(0.718163997970498,1.61508042700263,0.695997784676728));
#7072=CARTESIAN_POINT('Ctrl Pts',(0.713525491562421,1.5815373526696,0.700629269222037));
#7073=CARTESIAN_POINT('Ctrl Pts',(0.713525491562421,1.5184626473304,0.700629269222037));
#7074=CARTESIAN_POINT('Ctrl Pts',(0.718163997970498,1.48491957299737,0.695997784676728));
#7075=CARTESIAN_POINT('Ctrl Pts',(0.73619249062986,1.42336732874239,0.676899590973058));
#7076=CARTESIAN_POINT('Ctrl Pts',(0.749495710301794,1.39534588636318,0.662390652284073));
#7077=CARTESIAN_POINT('Ctrl Pts',(0.778498278845144,1.35110381617461,0.62804895077401));
#7078=CARTESIAN_POINT('Ctrl Pts',(0.796153444118959,1.33188468517318,0.605884303066698));
#7079=CARTESIAN_POINT('Ctrl Pts',(0.832065554235658,1.30632915724249,0.555538485325664));
#7080=CARTESIAN_POINT('Ctrl Pts',(0.850258932191534,1.3,0.527308329855003));
#7081=CARTESIAN_POINT('Ctrl Pts',(0.881791875377343,1.3,0.472691670144998));
#7082=CARTESIAN_POINT('Ctrl Pts',(0.897143218189782,1.30632915724249,0.442820664919227));
#7083=CARTESIAN_POINT('Ctrl Pts',(0.92278792026947,1.33188468517318,0.386546956384144));
#7084=CARTESIAN_POINT('Ctrl Pts',(0.933155485613026,1.35110381617461,0.360174810895352));
#7085=CARTESIAN_POINT('Ctrl Pts',(0.948394987258249,1.39534588636318,0.31788699900678));
#7086=CARTESIAN_POINT('Ctrl Pts',(0.954308486908894,1.42336732874239,0.299111603474268));
#7087=CARTESIAN_POINT('Ctrl Pts',(0.961833761492987,1.48491957299738,0.273949373987484));
#7088=CARTESIAN_POINT('Ctrl Pts',(0.963525491562421,1.5184626473304,0.267616567329818));
#7089=CARTESIAN_POINT('Ctrl Pts',(0.963525491562421,1.55,0.267616567329818));
#7090=CARTESIAN_POINT('Origin',(0.,1.55,0.));
#7091=CARTESIAN_POINT('',(-0.713525491562421,1.55,-0.700629269222037));
#7092=CARTESIAN_POINT('Ctrl Pts',(-0.713525491562421,1.55,-0.700629269222037));
#7093=CARTESIAN_POINT('Ctrl Pts',(-0.713525491562421,1.5184626473304,-0.700629269222037));
#7094=CARTESIAN_POINT('Ctrl Pts',(-0.718163997970498,1.48491957299737,-0.695997784676728));
#7095=CARTESIAN_POINT('Ctrl Pts',(-0.73619249062986,1.42336732874239,-0.676899590973058));
#7096=CARTESIAN_POINT('Ctrl Pts',(-0.749495710301794,1.39534588636318,-0.662390652284073));
#7097=CARTESIAN_POINT('Ctrl Pts',(-0.778498278845144,1.35110381617461,-0.62804895077401));
#7098=CARTESIAN_POINT('Ctrl Pts',(-0.796153444118959,1.33188468517318,-0.605884303066698));
#7099=CARTESIAN_POINT('Ctrl Pts',(-0.832065554235658,1.30632915724249,-0.555538485325664));
#7100=CARTESIAN_POINT('Ctrl Pts',(-0.850258932191534,1.3,-0.527308329855003));
#7101=CARTESIAN_POINT('Ctrl Pts',(-0.881791875377343,1.3,-0.472691670144998));
#7102=CARTESIAN_POINT('Ctrl Pts',(-0.897143218189782,1.30632915724249,-0.442820664919227));
#7103=CARTESIAN_POINT('Ctrl Pts',(-0.92278792026947,1.33188468517318,-0.386546956384144));
#7104=CARTESIAN_POINT('Ctrl Pts',(-0.933155485613026,1.35110381617461,-0.360174810895352));
#7105=CARTESIAN_POINT('Ctrl Pts',(-0.948394987258249,1.39534588636318,-0.31788699900678));
#7106=CARTESIAN_POINT('Ctrl Pts',(-0.954308486908894,1.42336732874239,-0.299111603474268));
#7107=CARTESIAN_POINT('Ctrl Pts',(-0.961833761492986,1.48491957299737,-0.273949373987484));
#7108=CARTESIAN_POINT('Ctrl Pts',(-0.963525491562421,1.5184626473304,-0.267616567329818));
#7109=CARTESIAN_POINT('Ctrl Pts',(-0.963525491562421,1.5815373526696,-0.267616567329818));
#7110=CARTESIAN_POINT('Ctrl Pts',(-0.961833761492986,1.61508042700263,-0.273949373987484));
#7111=CARTESIAN_POINT('Ctrl Pts',(-0.954308486908894,1.67663267125761,-0.299111603474268));
#7112=CARTESIAN_POINT('Ctrl Pts',(-0.948394987258249,1.70465411363682,-0.31788699900678));
#7113=CARTESIAN_POINT('Ctrl Pts',(-0.933155485613026,1.74889618382539,-0.360174810895352));
#7114=CARTESIAN_POINT('Ctrl Pts',(-0.92278792026947,1.76811531482682,-0.386546956384144));
#7115=CARTESIAN_POINT('Ctrl Pts',(-0.897143218189782,1.79367084275751,-0.442820664919227));
#7116=CARTESIAN_POINT('Ctrl Pts',(-0.881791875377343,1.8,-0.472691670144998));
#7117=CARTESIAN_POINT('Ctrl Pts',(-0.850258932191534,1.8,-0.527308329855003));
#7118=CARTESIAN_POINT('Ctrl Pts',(-0.832065554235658,1.79367084275751,-0.555538485325664));
#7119=CARTESIAN_POINT('Ctrl Pts',(-0.796153444118959,1.76811531482682,-0.605884303066698));
#7120=CARTESIAN_POINT('Ctrl Pts',(-0.778498278845144,1.74889618382539,-0.62804895077401));
#7121=CARTESIAN_POINT('Ctrl Pts',(-0.749495710301794,1.70465411363682,-0.662390652284073));
#7122=CARTESIAN_POINT('Ctrl Pts',(-0.73619249062986,1.67663267125761,-0.676899590973058));
#7123=CARTESIAN_POINT('Ctrl Pts',(-0.718163997970498,1.61508042700263,-0.695997784676728));
#7124=CARTESIAN_POINT('Ctrl Pts',(-0.713525491562421,1.5815373526696,-0.700629269222037));
#7125=CARTESIAN_POINT('Ctrl Pts',(-0.713525491562421,1.55,-0.700629269222037));
#7126=CARTESIAN_POINT('',(-1.28744468918255,1.55,-1.03198167246111));
#7127=CARTESIAN_POINT('',(0.125,1.55,-0.21650635094611));
#7128=CARTESIAN_POINT('',(-1.42894191624432,1.3,-0.825000000000001));
#7129=CARTESIAN_POINT('Ctrl Pts',(-1.42894191624432,1.3,-0.825000000000001));
#7130=CARTESIAN_POINT('Ctrl Pts',(-1.4132207435299,1.3,-0.852229869895949));
#7131=CARTESIAN_POINT('Ctrl Pts',(-1.39561049050871,1.30629366210296,-0.880751161609749));
#7132=CARTESIAN_POINT('Ctrl Pts',(-1.36172049302549,1.33182222741682,-0.932292094146256));
#7133=CARTESIAN_POINT('Ctrl Pts',(-1.34548213209931,1.35105447038507,-0.955340251466735));
#7134=CARTESIAN_POINT('Ctrl Pts',(-1.31917543061769,1.39539254159618,-0.991349264982991));
#7135=CARTESIAN_POINT('Ctrl Pts',(-1.30734972067592,1.42347183818157,-1.00672880483252));
#7136=CARTESIAN_POINT('Ctrl Pts',(-1.29146042158868,1.48505200040818,-1.02703269653942));
#7137=CARTESIAN_POINT('Ctrl Pts',(-1.28744468918255,1.51855708359447,-1.03198167246111));
#7138=CARTESIAN_POINT('Ctrl Pts',(-1.28744468918255,1.55,-1.03198167246111));
#7139=CARTESIAN_POINT('',(-1.42894191624432,1.8,-0.825000000000001));
#7140=CARTESIAN_POINT('Ctrl Pts',(-1.42894191624432,1.8,-0.825000000000001));
#7141=CARTESIAN_POINT('Ctrl Pts',(-1.44466308895875,1.8,-0.797770130104052));
#7142=CARTESIAN_POINT('Ctrl Pts',(-1.46055812562105,1.79370633789704,-0.768258557763732));
#7143=CARTESIAN_POINT('Ctrl Pts',(-1.48824888379079,1.76817777258318,-0.713138492740816));
#7144=CARTESIAN_POINT('Ctrl Pts',(-1.50008999307766,1.74894552961493,-0.687551581002689));
#7145=CARTESIAN_POINT('Ctrl Pts',(-1.51812136280714,1.70460745840382,-0.646764802471699));
#7146=CARTESIAN_POINT('Ctrl Pts',(-1.52552758004446,1.67652816181843,-0.628833667319578));
#7147=CARTESIAN_POINT('Ctrl Pts',(-1.53516661651472,1.61494799959182,-0.60492118480825));
#7148=CARTESIAN_POINT('Ctrl Pts',(-1.53744468918255,1.58144291640553,-0.598968970568896));
#7149=CARTESIAN_POINT('Ctrl Pts',(-1.53744468918255,1.51855708359447,-0.598968970568896));
#7150=CARTESIAN_POINT('Ctrl Pts',(-1.53516661651472,1.48505200040818,-0.60492118480825));
#7151=CARTESIAN_POINT('Ctrl Pts',(-1.52552758004446,1.42347183818157,-0.628833667319578));
#7152=CARTESIAN_POINT('Ctrl Pts',(-1.51812136280714,1.39539254159618,-0.646764802471699));
#7153=CARTESIAN_POINT('Ctrl Pts',(-1.50008999307766,1.35105447038507,-0.687551581002689));
#7154=CARTESIAN_POINT('Ctrl Pts',(-1.48824888379079,1.33182222741682,-0.713138492740816));
#7155=CARTESIAN_POINT('Ctrl Pts',(-1.46055812562105,1.30629366210296,-0.768258557763732));
#7156=CARTESIAN_POINT('Ctrl Pts',(-1.44466308895875,1.3,-0.797770130104052));
#7157=CARTESIAN_POINT('Ctrl Pts',(-1.42894191624432,1.3,-0.825000000000001));
#7158=CARTESIAN_POINT('Ctrl Pts',(-1.28744468918255,1.55,-1.03198167246111));
#7159=CARTESIAN_POINT('Ctrl Pts',(-1.28744468918255,1.58144291640553,-1.03198167246111));
#7160=CARTESIAN_POINT('Ctrl Pts',(-1.29146042158868,1.61494799959182,-1.02703269653942));
#7161=CARTESIAN_POINT('Ctrl Pts',(-1.30734972067592,1.67652816181843,-1.00672880483252));
#7162=CARTESIAN_POINT('Ctrl Pts',(-1.31917543061769,1.70460745840382,-0.991349264982991));
#7163=CARTESIAN_POINT('Ctrl Pts',(-1.34548213209931,1.74894552961493,-0.955340251466734));
#7164=CARTESIAN_POINT('Ctrl Pts',(-1.36172049302549,1.76817777258318,-0.932292094146256));
#7165=CARTESIAN_POINT('Ctrl Pts',(-1.39561049050871,1.79370633789704,-0.880751161609749));
#7166=CARTESIAN_POINT('Ctrl Pts',(-1.4132207435299,1.8,-0.852229869895949));
#7167=CARTESIAN_POINT('Ctrl Pts',(-1.42894191624432,1.8,-0.825000000000001));
#7168=CARTESIAN_POINT('Origin',(0.,1.55,0.));
#7169=CARTESIAN_POINT('',(-1.65,0.85,-2.02066721859313E-16));
#7170=CARTESIAN_POINT('Origin',(0.,0.85,0.));
#7171=CARTESIAN_POINT('',(-1.65,2.25,-2.02066721859313E-16));
#7172=CARTESIAN_POINT('',(-1.65,1.55,-2.02066721859313E-16));
#7173=CARTESIAN_POINT('Origin',(0.,2.25,0.));
#7174=CARTESIAN_POINT('',(-1.42894191624432,1.3,0.825));
#7175=CARTESIAN_POINT('',(-1.42894191624432,1.8,0.825));
#7176=CARTESIAN_POINT('Ctrl Pts',(-1.42894191624432,1.3,0.825));
#7177=CARTESIAN_POINT('Ctrl Pts',(-1.44466308895875,1.3,0.797770130104051));
#7178=CARTESIAN_POINT('Ctrl Pts',(-1.46055812562105,1.30629366210296,0.768258557763731));
#7179=CARTESIAN_POINT('Ctrl Pts',(-1.48824888379079,1.33182222741682,0.713138492740815));
#7180=CARTESIAN_POINT('Ctrl Pts',(-1.50008999307766,1.35105447038507,0.687551581002688));
#7181=CARTESIAN_POINT('Ctrl Pts',(-1.51812136280714,1.39539254159618,0.646764802471698));
#7182=CARTESIAN_POINT('Ctrl Pts',(-1.52552758004446,1.42347183818157,0.628833667319577));
#7183=CARTESIAN_POINT('Ctrl Pts',(-1.53516661651472,1.48505200040818,0.604921184808249));
#7184=CARTESIAN_POINT('Ctrl Pts',(-1.53744468918255,1.51855708359447,0.598968970568895));
#7185=CARTESIAN_POINT('Ctrl Pts',(-1.53744468918255,1.58144291640553,0.598968970568895));
#7186=CARTESIAN_POINT('Ctrl Pts',(-1.53516661651472,1.61494799959182,0.604921184808249));
#7187=CARTESIAN_POINT('Ctrl Pts',(-1.52552758004446,1.67652816181843,0.628833667319577));
#7188=CARTESIAN_POINT('Ctrl Pts',(-1.51812136280714,1.70460745840382,0.646764802471698));
#7189=CARTESIAN_POINT('Ctrl Pts',(-1.50008999307766,1.74894552961493,0.687551581002688));
#7190=CARTESIAN_POINT('Ctrl Pts',(-1.48824888379079,1.76817777258318,0.713138492740815));
#7191=CARTESIAN_POINT('Ctrl Pts',(-1.46055812562105,1.79370633789704,0.768258557763731));
#7192=CARTESIAN_POINT('Ctrl Pts',(-1.44466308895875,1.8,0.797770130104051));
#7193=CARTESIAN_POINT('Ctrl Pts',(-1.42894191624432,1.8,0.825));
#7194=CARTESIAN_POINT('',(-1.28744468918255,1.55,1.03198167246111));
#7195=CARTESIAN_POINT('Ctrl Pts',(-1.42894191624432,1.8,0.825));
#7196=CARTESIAN_POINT('Ctrl Pts',(-1.4132207435299,1.8,0.852229869895948));
#7197=CARTESIAN_POINT('Ctrl Pts',(-1.39561049050871,1.79370633789704,0.880751161609747));
#7198=CARTESIAN_POINT('Ctrl Pts',(-1.36172049302549,1.76817777258318,0.932292094146255));
#7199=CARTESIAN_POINT('Ctrl Pts',(-1.34548213209931,1.74894552961493,0.955340251466733));
#7200=CARTESIAN_POINT('Ctrl Pts',(-1.31917543061769,1.70460745840382,0.991349264982989));
#7201=CARTESIAN_POINT('Ctrl Pts',(-1.30734972067592,1.67652816181843,1.00672880483252));
#7202=CARTESIAN_POINT('Ctrl Pts',(-1.29146042158868,1.61494799959182,1.02703269653942));
#7203=CARTESIAN_POINT('Ctrl Pts',(-1.28744468918255,1.58144291640553,1.03198167246111));
#7204=CARTESIAN_POINT('Ctrl Pts',(-1.28744468918255,1.55,1.03198167246111));
#7205=CARTESIAN_POINT('Ctrl Pts',(-1.28744468918255,1.55,1.03198167246111));
#7206=CARTESIAN_POINT('Ctrl Pts',(-1.28744468918255,1.51855708359447,1.03198167246111));
#7207=CARTESIAN_POINT('Ctrl Pts',(-1.29146042158868,1.48505200040818,1.02703269653942));
#7208=CARTESIAN_POINT('Ctrl Pts',(-1.30734972067592,1.42347183818157,1.00672880483252));
#7209=CARTESIAN_POINT('Ctrl Pts',(-1.31917543061769,1.39539254159618,0.99134926498299));
#7210=CARTESIAN_POINT('Ctrl Pts',(-1.34548213209931,1.35105447038508,0.955340251466733));
#7211=CARTESIAN_POINT('Ctrl Pts',(-1.36172049302549,1.33182222741682,0.932292094146255));
#7212=CARTESIAN_POINT('Ctrl Pts',(-1.39561049050871,1.30629366210296,0.880751161609748));
#7213=CARTESIAN_POINT('Ctrl Pts',(-1.4132207435299,1.3,0.852229869895949));
#7214=CARTESIAN_POINT('Ctrl Pts',(-1.42894191624432,1.3,0.825));
#7215=CARTESIAN_POINT('',(1.42894191624432,1.8,-0.825));
#7216=CARTESIAN_POINT('',(1.42894191624432,1.3,-0.825));
#7217=CARTESIAN_POINT('Ctrl Pts',(1.42894191624432,1.8,-0.825));
#7218=CARTESIAN_POINT('Ctrl Pts',(1.4132207435299,1.8,-0.852229869895949));
#7219=CARTESIAN_POINT('Ctrl Pts',(1.39561049050871,1.79370633789704,-0.880751161609748));
#7220=CARTESIAN_POINT('Ctrl Pts',(1.36172049302549,1.76817777258318,-0.932292094146255));
#7221=CARTESIAN_POINT('Ctrl Pts',(1.34548213209931,1.74894552961493,-0.955340251466734));
#7222=CARTESIAN_POINT('Ctrl Pts',(1.31917543061769,1.70460745840382,-0.99134926498299));
#7223=CARTESIAN_POINT('Ctrl Pts',(1.30734972067592,1.67652816181843,-1.00672880483252));
#7224=CARTESIAN_POINT('Ctrl Pts',(1.29146042158868,1.61494799959182,-1.02703269653942));
#7225=CARTESIAN_POINT('Ctrl Pts',(1.28744468918255,1.58144291640553,-1.03198167246111));
#7226=CARTESIAN_POINT('Ctrl Pts',(1.28744468918255,1.51855708359447,-1.03198167246111));
#7227=CARTESIAN_POINT('Ctrl Pts',(1.29146042158868,1.48505200040818,-1.02703269653942));
#7228=CARTESIAN_POINT('Ctrl Pts',(1.30734972067592,1.42347183818157,-1.00672880483252));
#7229=CARTESIAN_POINT('Ctrl Pts',(1.31917543061769,1.39539254159618,-0.99134926498299));
#7230=CARTESIAN_POINT('Ctrl Pts',(1.34548213209931,1.35105447038507,-0.955340251466734));
#7231=CARTESIAN_POINT('Ctrl Pts',(1.36172049302549,1.33182222741682,-0.932292094146255));
#7232=CARTESIAN_POINT('Ctrl Pts',(1.39561049050871,1.30629366210296,-0.880751161609748));
#7233=CARTESIAN_POINT('Ctrl Pts',(1.4132207435299,1.3,-0.852229869895948));
#7234=CARTESIAN_POINT('Ctrl Pts',(1.42894191624432,1.3,-0.825));
#7235=CARTESIAN_POINT('',(1.53744468918255,1.55,-0.598968970568895));
#7236=CARTESIAN_POINT('Ctrl Pts',(1.42894191624432,1.3,-0.825));
#7237=CARTESIAN_POINT('Ctrl Pts',(1.44466308895875,1.3,-0.797770130104051));
#7238=CARTESIAN_POINT('Ctrl Pts',(1.46055812562105,1.30629366210296,-0.768258557763731));
#7239=CARTESIAN_POINT('Ctrl Pts',(1.48824888379079,1.33182222741682,-0.713138492740815));
#7240=CARTESIAN_POINT('Ctrl Pts',(1.50008999307766,1.35105447038507,-0.687551581002688));
#7241=CARTESIAN_POINT('Ctrl Pts',(1.51812136280714,1.39539254159618,-0.646764802471698));
#7242=CARTESIAN_POINT('Ctrl Pts',(1.52552758004446,1.42347183818157,-0.628833667319577));
#7243=CARTESIAN_POINT('Ctrl Pts',(1.53516661651472,1.48505200040818,-0.604921184808249));
#7244=CARTESIAN_POINT('Ctrl Pts',(1.53744468918255,1.51855708359447,-0.598968970568895));
#7245=CARTESIAN_POINT('Ctrl Pts',(1.53744468918255,1.55,-0.598968970568895));
#7246=CARTESIAN_POINT('Ctrl Pts',(1.53744468918255,1.55,-0.598968970568895));
#7247=CARTESIAN_POINT('Ctrl Pts',(1.53744468918255,1.58144291640553,-0.598968970568895));
#7248=CARTESIAN_POINT('Ctrl Pts',(1.53516661651472,1.61494799959182,-0.604921184808249));
#7249=CARTESIAN_POINT('Ctrl Pts',(1.52552758004446,1.67652816181843,-0.628833667319577));
#7250=CARTESIAN_POINT('Ctrl Pts',(1.51812136280714,1.70460745840382,-0.646764802471698));
#7251=CARTESIAN_POINT('Ctrl Pts',(1.50008999307766,1.74894552961493,-0.687551581002688));
#7252=CARTESIAN_POINT('Ctrl Pts',(1.48824888379079,1.76817777258318,-0.713138492740815));
#7253=CARTESIAN_POINT('Ctrl Pts',(1.46055812562105,1.79370633789704,-0.768258557763731));
#7254=CARTESIAN_POINT('Ctrl Pts',(1.44466308895875,1.8,-0.797770130104051));
#7255=CARTESIAN_POINT('Ctrl Pts',(1.42894191624432,1.8,-0.825));
#7256=CARTESIAN_POINT('',(0.,1.3,-1.65));
#7257=CARTESIAN_POINT('',(0.,1.8,-1.65));
#7258=CARTESIAN_POINT('Ctrl Pts',(1.38777878078145E-17,1.3,-1.65));
#7259=CARTESIAN_POINT('Ctrl Pts',(0.0314423454288489,1.3,-1.65));
#7260=CARTESIAN_POINT('Ctrl Pts',(0.0649476351123396,1.30629366210296,-1.64900971937348));
#7261=CARTESIAN_POINT('Ctrl Pts',(0.126528390765307,1.33182222741682,-1.64543058688707));
#7262=CARTESIAN_POINT('Ctrl Pts',(0.154607860978348,1.35105447038507,-1.64289183246942));
#7263=CARTESIAN_POINT('Ctrl Pts',(0.198945932189457,1.39539254159618,-1.63811406745469));
#7264=CARTESIAN_POINT('Ctrl Pts',(0.218177859368546,1.42347183818157,-1.63556247215209));
#7265=CARTESIAN_POINT('Ctrl Pts',(0.243706194926033,1.48505200040818,-1.63195388134767));
#7266=CARTESIAN_POINT('Ctrl Pts',(0.25,1.51855708359447,-1.63095064303001));
#7267=CARTESIAN_POINT('Ctrl Pts',(0.25,1.58144291640553,-1.63095064303001));
#7268=CARTESIAN_POINT('Ctrl Pts',(0.243706194926033,1.61494799959182,-1.63195388134767));
#7269=CARTESIAN_POINT('Ctrl Pts',(0.218177859368546,1.67652816181843,-1.63556247215209));
#7270=CARTESIAN_POINT('Ctrl Pts',(0.198945932189457,1.70460745840382,-1.63811406745469));
#7271=CARTESIAN_POINT('Ctrl Pts',(0.154607860978349,1.74894552961493,-1.64289183246942));
#7272=CARTESIAN_POINT('Ctrl Pts',(0.126528390765307,1.76817777258318,-1.64543058688707));
#7273=CARTESIAN_POINT('Ctrl Pts',(0.0649476351123398,1.79370633789704,-1.64900971937348));
#7274=CARTESIAN_POINT('Ctrl Pts',(0.031442345428849,1.8,-1.65));
#7275=CARTESIAN_POINT('Ctrl Pts',(7.63278329429795E-17,1.8,-1.65));
#7276=CARTESIAN_POINT('',(-0.25,1.55,-1.63095064303001));
#7277=CARTESIAN_POINT('Ctrl Pts',(9.0205620750794E-17,1.8,-1.65));
#7278=CARTESIAN_POINT('Ctrl Pts',(-0.0314423454288488,1.8,-1.65));
#7279=CARTESIAN_POINT('Ctrl Pts',(-0.0649476351123396,1.79370633789704,
-1.64900971937348));
#7280=CARTESIAN_POINT('Ctrl Pts',(-0.126528390765307,1.76817777258318,-1.64543058688707));
#7281=CARTESIAN_POINT('Ctrl Pts',(-0.154607860978348,1.74894552961493,-1.64289183246942));
#7282=CARTESIAN_POINT('Ctrl Pts',(-0.198945932189456,1.70460745840382,-1.63811406745469));
#7283=CARTESIAN_POINT('Ctrl Pts',(-0.218177859368546,1.67652816181843,-1.63556247215209));
#7284=CARTESIAN_POINT('Ctrl Pts',(-0.243706194926033,1.61494799959182,-1.63195388134767));
#7285=CARTESIAN_POINT('Ctrl Pts',(-0.25,1.58144291640553,-1.63095064303001));
#7286=CARTESIAN_POINT('Ctrl Pts',(-0.25,1.55,-1.63095064303001));
#7287=CARTESIAN_POINT('Ctrl Pts',(-0.25,1.55,-1.63095064303001));
#7288=CARTESIAN_POINT('Ctrl Pts',(-0.25,1.51855708359447,-1.63095064303001));
#7289=CARTESIAN_POINT('Ctrl Pts',(-0.243706194926033,1.48505200040818,-1.63195388134767));
#7290=CARTESIAN_POINT('Ctrl Pts',(-0.218177859368546,1.42347183818157,-1.63556247215209));
#7291=CARTESIAN_POINT('Ctrl Pts',(-0.198945932189457,1.39539254159618,-1.63811406745469));
#7292=CARTESIAN_POINT('Ctrl Pts',(-0.154607860978349,1.35105447038507,-1.64289183246942));
#7293=CARTESIAN_POINT('Ctrl Pts',(-0.126528390765307,1.33182222741682,-1.64543058688707));
#7294=CARTESIAN_POINT('Ctrl Pts',(-0.0649476351123398,1.30629366210296,
-1.64900971937348));
#7295=CARTESIAN_POINT('Ctrl Pts',(-0.031442345428849,1.3,-1.65));
#7296=CARTESIAN_POINT('Ctrl Pts',(-4.85722573273506E-17,1.3,-1.65));
#7297=CARTESIAN_POINT('',(0.,1.8,1.65));
#7298=CARTESIAN_POINT('',(0.,1.3,1.65));
#7299=CARTESIAN_POINT('Ctrl Pts',(8.32667268468867E-17,1.8,1.65));
#7300=CARTESIAN_POINT('Ctrl Pts',(0.031442345428849,1.8,1.65));
#7301=CARTESIAN_POINT('Ctrl Pts',(0.0649476351123398,1.79370633789704,1.64900971937348));
#7302=CARTESIAN_POINT('Ctrl Pts',(0.126528390765307,1.76817777258318,1.64543058688707));
#7303=CARTESIAN_POINT('Ctrl Pts',(0.154607860978349,1.74894552961493,1.64289183246942));
#7304=CARTESIAN_POINT('Ctrl Pts',(0.198945932189457,1.70460745840382,1.63811406745469));
#7305=CARTESIAN_POINT('Ctrl Pts',(0.218177859368546,1.67652816181843,1.63556247215209));
#7306=CARTESIAN_POINT('Ctrl Pts',(0.243706194926033,1.61494799959182,1.63195388134767));
#7307=CARTESIAN_POINT('Ctrl Pts',(0.25,1.58144291640553,1.63095064303001));
#7308=CARTESIAN_POINT('Ctrl Pts',(0.25,1.51855708359447,1.63095064303001));
#7309=CARTESIAN_POINT('Ctrl Pts',(0.243706194926033,1.48505200040818,1.63195388134767));
#7310=CARTESIAN_POINT('Ctrl Pts',(0.218177859368546,1.42347183818157,1.63556247215209));
#7311=CARTESIAN_POINT('Ctrl Pts',(0.198945932189457,1.39539254159618,1.63811406745469));
#7312=CARTESIAN_POINT('Ctrl Pts',(0.154607860978348,1.35105447038507,1.64289183246942));
#7313=CARTESIAN_POINT('Ctrl Pts',(0.126528390765307,1.33182222741682,1.64543058688707));
#7314=CARTESIAN_POINT('Ctrl Pts',(0.0649476351123397,1.30629366210296,1.64900971937348));
#7315=CARTESIAN_POINT('Ctrl Pts',(0.0314423454288488,1.3,1.65));
#7316=CARTESIAN_POINT('Ctrl Pts',(-1.38777878078145E-17,1.3,1.65));
#7317=CARTESIAN_POINT('',(-0.25,1.55,1.63095064303001));
#7318=CARTESIAN_POINT('Ctrl Pts',(-5.55111512312578E-17,1.3,1.65));
#7319=CARTESIAN_POINT('Ctrl Pts',(-0.031442345428849,1.3,1.65));
#7320=CARTESIAN_POINT('Ctrl Pts',(-0.0649476351123398,1.30629366210296,
1.64900971937348));
#7321=CARTESIAN_POINT('Ctrl Pts',(-0.126528390765307,1.33182222741682,1.64543058688707));
#7322=CARTESIAN_POINT('Ctrl Pts',(-0.154607860978349,1.35105447038507,1.64289183246942));
#7323=CARTESIAN_POINT('Ctrl Pts',(-0.198945932189457,1.39539254159618,1.63811406745469));
#7324=CARTESIAN_POINT('Ctrl Pts',(-0.218177859368546,1.42347183818157,1.63556247215209));
#7325=CARTESIAN_POINT('Ctrl Pts',(-0.243706194926033,1.48505200040818,1.63195388134767));
#7326=CARTESIAN_POINT('Ctrl Pts',(-0.25,1.51855708359447,1.63095064303001));
#7327=CARTESIAN_POINT('Ctrl Pts',(-0.25,1.55,1.63095064303001));
#7328=CARTESIAN_POINT('Ctrl Pts',(-0.25,1.55,1.63095064303001));
#7329=CARTESIAN_POINT('Ctrl Pts',(-0.25,1.58144291640553,1.63095064303001));
#7330=CARTESIAN_POINT('Ctrl Pts',(-0.243706194926033,1.61494799959182,1.63195388134767));
#7331=CARTESIAN_POINT('Ctrl Pts',(-0.218177859368546,1.67652816181843,1.63556247215209));
#7332=CARTESIAN_POINT('Ctrl Pts',(-0.198945932189456,1.70460745840382,1.63811406745469));
#7333=CARTESIAN_POINT('Ctrl Pts',(-0.154607860978348,1.74894552961493,1.64289183246942));
#7334=CARTESIAN_POINT('Ctrl Pts',(-0.126528390765307,1.76817777258318,1.64543058688707));
#7335=CARTESIAN_POINT('Ctrl Pts',(-0.0649476351123396,1.79370633789704,
1.64900971937348));
#7336=CARTESIAN_POINT('Ctrl Pts',(-0.0314423454288488,1.8,1.65));
#7337=CARTESIAN_POINT('Ctrl Pts',(7.63278329429795E-17,1.8,1.65));
#7338=CARTESIAN_POINT('Origin',(0.,1.55,0.));
#7339=CARTESIAN_POINT('',(-0.713525491562421,1.55,0.700629269222037));
#7340=CARTESIAN_POINT('',(0.125,1.55,0.21650635094611));
#7341=CARTESIAN_POINT('Ctrl Pts',(-0.713525491562421,1.55,0.700629269222037));
#7342=CARTESIAN_POINT('Ctrl Pts',(-0.713525491562421,1.5815373526696,0.700629269222037));
#7343=CARTESIAN_POINT('Ctrl Pts',(-0.718163997970498,1.61508042700263,0.695997784676727));
#7344=CARTESIAN_POINT('Ctrl Pts',(-0.73619249062986,1.67663267125761,0.676899590973058));
#7345=CARTESIAN_POINT('Ctrl Pts',(-0.749495710301795,1.70465411363682,0.662390652284073));
#7346=CARTESIAN_POINT('Ctrl Pts',(-0.778498278845144,1.74889618382539,0.628048950774009));
#7347=CARTESIAN_POINT('Ctrl Pts',(-0.796153444118959,1.76811531482682,0.605884303066698));
#7348=CARTESIAN_POINT('Ctrl Pts',(-0.832065554235658,1.79367084275751,0.555538485325663));
#7349=CARTESIAN_POINT('Ctrl Pts',(-0.850258932191534,1.8,0.527308329855002));
#7350=CARTESIAN_POINT('Ctrl Pts',(-0.881791875377343,1.8,0.472691670144998));
#7351=CARTESIAN_POINT('Ctrl Pts',(-0.897143218189782,1.79367084275751,0.442820664919227));
#7352=CARTESIAN_POINT('Ctrl Pts',(-0.92278792026947,1.76811531482682,0.386546956384144));
#7353=CARTESIAN_POINT('Ctrl Pts',(-0.933155485613026,1.74889618382539,0.360174810895352));
#7354=CARTESIAN_POINT('Ctrl Pts',(-0.948394987258249,1.70465411363682,0.31788699900678));
#7355=CARTESIAN_POINT('Ctrl Pts',(-0.954308486908894,1.67663267125761,0.299111603474267));
#7356=CARTESIAN_POINT('Ctrl Pts',(-0.961833761492987,1.61508042700263,0.273949373987484));
#7357=CARTESIAN_POINT('Ctrl Pts',(-0.963525491562421,1.5815373526696,0.267616567329817));
#7358=CARTESIAN_POINT('Ctrl Pts',(-0.963525491562421,1.5184626473304,0.267616567329817));
#7359=CARTESIAN_POINT('Ctrl Pts',(-0.961833761492987,1.48491957299737,0.273949373987484));
#7360=CARTESIAN_POINT('Ctrl Pts',(-0.954308486908894,1.42336732874239,0.299111603474267));
#7361=CARTESIAN_POINT('Ctrl Pts',(-0.948394987258249,1.39534588636318,0.31788699900678));
#7362=CARTESIAN_POINT('Ctrl Pts',(-0.933155485613026,1.35110381617461,0.360174810895352));
#7363=CARTESIAN_POINT('Ctrl Pts',(-0.92278792026947,1.33188468517318,0.386546956384144));
#7364=CARTESIAN_POINT('Ctrl Pts',(-0.897143218189782,1.30632915724249,0.442820664919227));
#7365=CARTESIAN_POINT('Ctrl Pts',(-0.881791875377343,1.3,0.472691670144998));
#7366=CARTESIAN_POINT('Ctrl Pts',(-0.850258932191534,1.3,0.527308329855002));
#7367=CARTESIAN_POINT('Ctrl Pts',(-0.832065554235658,1.30632915724249,0.555538485325663));
#7368=CARTESIAN_POINT('Ctrl Pts',(-0.796153444118959,1.33188468517318,0.605884303066698));
#7369=CARTESIAN_POINT('Ctrl Pts',(-0.778498278845144,1.35110381617461,0.628048950774009));
#7370=CARTESIAN_POINT('Ctrl Pts',(-0.749495710301795,1.39534588636318,0.662390652284073));
#7371=CARTESIAN_POINT('Ctrl Pts',(-0.73619249062986,1.42336732874239,0.676899590973058));
#7372=CARTESIAN_POINT('Ctrl Pts',(-0.718163997970498,1.48491957299737,0.695997784676727));
#7373=CARTESIAN_POINT('Ctrl Pts',(-0.713525491562421,1.5184626473304,0.700629269222037));
#7374=CARTESIAN_POINT('Ctrl Pts',(-0.713525491562421,1.55,0.700629269222037));
#7375=CARTESIAN_POINT('Origin',(0.,1.55,0.));
#7376=CARTESIAN_POINT('',(0.963525491562421,1.55,-0.267616567329817));
#7377=CARTESIAN_POINT('Ctrl Pts',(0.963525491562421,1.55,-0.267616567329817));
#7378=CARTESIAN_POINT('Ctrl Pts',(0.963525491562421,1.5184626473304,-0.267616567329817));
#7379=CARTESIAN_POINT('Ctrl Pts',(0.961833761492987,1.48491957299737,-0.273949373987484));
#7380=CARTESIAN_POINT('Ctrl Pts',(0.954308486908894,1.42336732874239,-0.299111603474267));
#7381=CARTESIAN_POINT('Ctrl Pts',(0.948394987258249,1.39534588636318,-0.31788699900678));
#7382=CARTESIAN_POINT('Ctrl Pts',(0.933155485613026,1.35110381617461,-0.360174810895352));
#7383=CARTESIAN_POINT('Ctrl Pts',(0.92278792026947,1.33188468517318,-0.386546956384144));
#7384=CARTESIAN_POINT('Ctrl Pts',(0.897143218189782,1.30632915724249,-0.442820664919227));
#7385=CARTESIAN_POINT('Ctrl Pts',(0.881791875377343,1.3,-0.472691670144998));
#7386=CARTESIAN_POINT('Ctrl Pts',(0.850258932191534,1.3,-0.527308329855002));
#7387=CARTESIAN_POINT('Ctrl Pts',(0.832065554235658,1.30632915724249,-0.555538485325663));
#7388=CARTESIAN_POINT('Ctrl Pts',(0.796153444118959,1.33188468517318,-0.605884303066698));
#7389=CARTESIAN_POINT('Ctrl Pts',(0.778498278845144,1.35110381617461,-0.628048950774009));
#7390=CARTESIAN_POINT('Ctrl Pts',(0.749495710301795,1.39534588636318,-0.662390652284073));
#7391=CARTESIAN_POINT('Ctrl Pts',(0.73619249062986,1.42336732874239,-0.676899590973058));
#7392=CARTESIAN_POINT('Ctrl Pts',(0.718163997970498,1.48491957299737,-0.695997784676727));
#7393=CARTESIAN_POINT('Ctrl Pts',(0.713525491562421,1.5184626473304,-0.700629269222037));
#7394=CARTESIAN_POINT('Ctrl Pts',(0.713525491562421,1.5815373526696,-0.700629269222037));
#7395=CARTESIAN_POINT('Ctrl Pts',(0.718163997970498,1.61508042700263,-0.695997784676727));
#7396=CARTESIAN_POINT('Ctrl Pts',(0.73619249062986,1.67663267125761,-0.676899590973058));
#7397=CARTESIAN_POINT('Ctrl Pts',(0.749495710301795,1.70465411363682,-0.662390652284073));
#7398=CARTESIAN_POINT('Ctrl Pts',(0.778498278845144,1.74889618382539,-0.628048950774009));
#7399=CARTESIAN_POINT('Ctrl Pts',(0.796153444118959,1.76811531482682,-0.605884303066698));
#7400=CARTESIAN_POINT('Ctrl Pts',(0.832065554235658,1.79367084275751,-0.555538485325663));
#7401=CARTESIAN_POINT('Ctrl Pts',(0.850258932191534,1.8,-0.527308329855002));
#7402=CARTESIAN_POINT('Ctrl Pts',(0.881791875377343,1.8,-0.472691670144998));
#7403=CARTESIAN_POINT('Ctrl Pts',(0.897143218189782,1.79367084275751,-0.442820664919227));
#7404=CARTESIAN_POINT('Ctrl Pts',(0.92278792026947,1.76811531482682,-0.386546956384144));
#7405=CARTESIAN_POINT('Ctrl Pts',(0.933155485613026,1.74889618382539,-0.360174810895352));
#7406=CARTESIAN_POINT('Ctrl Pts',(0.948394987258249,1.70465411363682,-0.31788699900678));
#7407=CARTESIAN_POINT('Ctrl Pts',(0.954308486908894,1.67663267125761,-0.299111603474267));
#7408=CARTESIAN_POINT('Ctrl Pts',(0.961833761492987,1.61508042700263,-0.273949373987484));
#7409=CARTESIAN_POINT('Ctrl Pts',(0.963525491562421,1.5815373526696,-0.267616567329817));
#7410=CARTESIAN_POINT('Ctrl Pts',(0.963525491562421,1.55,-0.267616567329817));
#7411=CARTESIAN_POINT('',(0.125,1.55,0.21650635094611));
#7412=CARTESIAN_POINT('Origin',(0.,1.55,0.));
#7413=CARTESIAN_POINT('',(-0.25,1.55,-0.968245836551854));
#7414=CARTESIAN_POINT('',(-0.25,1.55,0.));
#7415=CARTESIAN_POINT('Ctrl Pts',(-0.25,1.55,-0.968245836551854));
#7416=CARTESIAN_POINT('Ctrl Pts',(-0.25,1.5815373526696,-0.968245836551854));
#7417=CARTESIAN_POINT('Ctrl Pts',(-0.243669763522489,1.61508042700263,-0.969947158664211));
#7418=CARTESIAN_POINT('Ctrl Pts',(-0.218115996279034,1.67663267125761,-0.976011194447325));
#7419=CARTESIAN_POINT('Ctrl Pts',(-0.198899276956455,1.70465411363682,-0.980277651290853));
#7420=CARTESIAN_POINT('Ctrl Pts',(-0.154657206767882,1.74889618382539,-0.988223761669361));
#7421=CARTESIAN_POINT('Ctrl Pts',(-0.126634476150511,1.76811531482682,-0.992431259450842));
#7422=CARTESIAN_POINT('Ctrl Pts',(-0.0650776639541238,1.79367084275751,
-0.99835915024489));
#7423=CARTESIAN_POINT('Ctrl Pts',(-0.0315329431858092,1.8,-1.));
#7424=CARTESIAN_POINT('Ctrl Pts',(0.0315329431858092,1.8,-1.));
#7425=CARTESIAN_POINT('Ctrl Pts',(0.0650776639541238,1.79367084275751,-0.99835915024489));
#7426=CARTESIAN_POINT('Ctrl Pts',(0.126634476150511,1.76811531482682,-0.992431259450842));
#7427=CARTESIAN_POINT('Ctrl Pts',(0.154657206767882,1.74889618382539,-0.988223761669361));
#7428=CARTESIAN_POINT('Ctrl Pts',(0.198899276956455,1.70465411363682,-0.980277651290853));
#7429=CARTESIAN_POINT('Ctrl Pts',(0.218115996279034,1.67663267125761,-0.976011194447325));
#7430=CARTESIAN_POINT('Ctrl Pts',(0.243669763522488,1.61508042700263,-0.969947158664211));
#7431=CARTESIAN_POINT('Ctrl Pts',(0.25,1.5815373526696,-0.968245836551854));
#7432=CARTESIAN_POINT('Ctrl Pts',(0.25,1.5184626473304,-0.968245836551854));
#7433=CARTESIAN_POINT('Ctrl Pts',(0.243669763522488,1.48491957299737,-0.969947158664211));
#7434=CARTESIAN_POINT('Ctrl Pts',(0.218115996279034,1.42336732874239,-0.976011194447325));
#7435=CARTESIAN_POINT('Ctrl Pts',(0.198899276956455,1.39534588636318,-0.980277651290853));
#7436=CARTESIAN_POINT('Ctrl Pts',(0.154657206767882,1.35110381617461,-0.988223761669361));
#7437=CARTESIAN_POINT('Ctrl Pts',(0.126634476150511,1.33188468517318,-0.992431259450842));
#7438=CARTESIAN_POINT('Ctrl Pts',(0.0650776639541239,1.30632915724249,-0.99835915024489));
#7439=CARTESIAN_POINT('Ctrl Pts',(0.0315329431858092,1.3,-1.));
#7440=CARTESIAN_POINT('Ctrl Pts',(-0.0315329431858092,1.3,-1.));
#7441=CARTESIAN_POINT('Ctrl Pts',(-0.0650776639541239,1.30632915724249,
-0.99835915024489));
#7442=CARTESIAN_POINT('Ctrl Pts',(-0.126634476150511,1.33188468517318,-0.992431259450842));
#7443=CARTESIAN_POINT('Ctrl Pts',(-0.154657206767882,1.35110381617461,-0.988223761669361));
#7444=CARTESIAN_POINT('Ctrl Pts',(-0.198899276956455,1.39534588636318,-0.980277651290853));
#7445=CARTESIAN_POINT('Ctrl Pts',(-0.218115996279034,1.42336732874239,-0.976011194447325));
#7446=CARTESIAN_POINT('Ctrl Pts',(-0.243669763522489,1.48491957299737,-0.969947158664211));
#7447=CARTESIAN_POINT('Ctrl Pts',(-0.25,1.5184626473304,-0.968245836551854));
#7448=CARTESIAN_POINT('Ctrl Pts',(-0.25,1.55,-0.968245836551854));
#7449=CARTESIAN_POINT('Origin',(0.,1.55,0.));
#7450=CARTESIAN_POINT('',(-0.25,1.55,0.968245836551854));
#7451=CARTESIAN_POINT('Ctrl Pts',(-0.25,1.55,0.968245836551854));
#7452=CARTESIAN_POINT('Ctrl Pts',(-0.25,1.5184626473304,0.968245836551854));
#7453=CARTESIAN_POINT('Ctrl Pts',(-0.243669763522489,1.48491957299737,0.969947158664211));
#7454=CARTESIAN_POINT('Ctrl Pts',(-0.218115996279034,1.42336732874239,0.976011194447325));
#7455=CARTESIAN_POINT('Ctrl Pts',(-0.198899276956455,1.39534588636318,0.980277651290853));
#7456=CARTESIAN_POINT('Ctrl Pts',(-0.154657206767882,1.35110381617461,0.988223761669361));
#7457=CARTESIAN_POINT('Ctrl Pts',(-0.126634476150511,1.33188468517318,0.992431259450842));
#7458=CARTESIAN_POINT('Ctrl Pts',(-0.065077663954124,1.30632915724249,0.99835915024489));
#7459=CARTESIAN_POINT('Ctrl Pts',(-0.0315329431858092,1.3,1.));
#7460=CARTESIAN_POINT('Ctrl Pts',(0.0315329431858092,1.3,1.));
#7461=CARTESIAN_POINT('Ctrl Pts',(0.065077663954124,1.30632915724249,0.99835915024489));
#7462=CARTESIAN_POINT('Ctrl Pts',(0.126634476150511,1.33188468517318,0.992431259450842));
#7463=CARTESIAN_POINT('Ctrl Pts',(0.154657206767882,1.35110381617461,0.988223761669361));
#7464=CARTESIAN_POINT('Ctrl Pts',(0.198899276956455,1.39534588636318,0.980277651290853));
#7465=CARTESIAN_POINT('Ctrl Pts',(0.218115996279034,1.42336732874239,0.976011194447325));
#7466=CARTESIAN_POINT('Ctrl Pts',(0.243669763522488,1.48491957299737,0.969947158664211));
#7467=CARTESIAN_POINT('Ctrl Pts',(0.25,1.5184626473304,0.968245836551854));
#7468=CARTESIAN_POINT('Ctrl Pts',(0.25,1.5815373526696,0.968245836551854));
#7469=CARTESIAN_POINT('Ctrl Pts',(0.243669763522488,1.61508042700263,0.969947158664211));
#7470=CARTESIAN_POINT('Ctrl Pts',(0.218115996279034,1.67663267125761,0.976011194447325));
#7471=CARTESIAN_POINT('Ctrl Pts',(0.198899276956455,1.70465411363682,0.980277651290853));
#7472=CARTESIAN_POINT('Ctrl Pts',(0.154657206767882,1.74889618382539,0.988223761669361));
#7473=CARTESIAN_POINT('Ctrl Pts',(0.126634476150511,1.76811531482682,0.992431259450842));
#7474=CARTESIAN_POINT('Ctrl Pts',(0.0650776639541239,1.79367084275751,0.99835915024489));
#7475=CARTESIAN_POINT('Ctrl Pts',(0.0315329431858092,1.8,1.));
#7476=CARTESIAN_POINT('Ctrl Pts',(-0.0315329431858092,1.8,1.));
#7477=CARTESIAN_POINT('Ctrl Pts',(-0.0650776639541239,1.79367084275751,
0.99835915024489));
#7478=CARTESIAN_POINT('Ctrl Pts',(-0.126634476150511,1.76811531482682,0.992431259450842));
#7479=CARTESIAN_POINT('Ctrl Pts',(-0.154657206767882,1.74889618382539,0.988223761669361));
#7480=CARTESIAN_POINT('Ctrl Pts',(-0.198899276956455,1.70465411363682,0.980277651290853));
#7481=CARTESIAN_POINT('Ctrl Pts',(-0.218115996279034,1.67663267125761,0.976011194447325));
#7482=CARTESIAN_POINT('Ctrl Pts',(-0.243669763522489,1.61508042700263,0.969947158664211));
#7483=CARTESIAN_POINT('Ctrl Pts',(-0.25,1.5815373526696,0.968245836551854));
#7484=CARTESIAN_POINT('Ctrl Pts',(-0.25,1.55,0.968245836551854));
#7485=CARTESIAN_POINT('',(-0.25,1.55,0.));
#7486=CARTESIAN_POINT('Origin',(1.65,2.25,0.));
#7487=CARTESIAN_POINT('',(-1.,2.25,-1.22464679914735E-16));
#7488=CARTESIAN_POINT('Origin',(0.,2.25,0.));
#7489=CARTESIAN_POINT('Origin',(1.75,0.85,0.));
#7490=CARTESIAN_POINT('',(-1.75,0.85,-2.14313189850787E-16));
#7491=CARTESIAN_POINT('Origin',(0.,0.85,0.));
#7492=CARTESIAN_POINT('Origin',(0.,0.,0.));
#7493=CARTESIAN_POINT('',(-1.75,-0.85,-2.14313189850787E-16));
#7494=CARTESIAN_POINT('Origin',(0.,-0.85,0.));
#7495=CARTESIAN_POINT('',(-1.75,0.,-2.14313189850787E-16));
#7496=CARTESIAN_POINT('Origin',(1.,-0.85,0.));
#7497=CARTESIAN_POINT('',(-1.,-0.85,-1.22464679914735E-16));
#7498=CARTESIAN_POINT('Origin',(0.,-0.85,0.));
#7499=CARTESIAN_POINT('Origin',(0.,0.7,0.));
#7500=CARTESIAN_POINT('',(-1.,0.7,-1.22464679914735E-16));
#8331=UNCERTAINTY_MEASURE_WITH_UNIT(LENGTH_MEASURE(0.001),#8378,
'DISTANCE_ACCURACY_VALUE',
'Maximum model space distance between geometric entities at asserted c
onnectivities');
#8345=UNCERTAINTY_MEASURE_WITH_UNIT(LENGTH_MEASURE(0.001),#8378,
'DISTANCE_ACCURACY_VALUE',
'Maximum model space distance between geometric entities at asserted c
onnectivities');
#8363=(
GEOMETRIC_REPRESENTATION_CONTEXT(3)
GLOBAL_UNCERTAINTY_ASSIGNED_CONTEXT((#8331))
GLOBAL_UNIT_ASSIGNED_CONTEXT((#8378,#8380,#8381))
REPRESENTATION_CONTEXT('','3D')
);
#8377=(
GEOMETRIC_REPRESENTATION_CONTEXT(3)
GLOBAL_UNCERTAINTY_ASSIGNED_CONTEXT((#8345))
GLOBAL_UNIT_ASSIGNED_CONTEXT((#8378,#8380,#8381))
REPRESENTATION_CONTEXT('','3D')
);
#8378=(
LENGTH_UNIT()
NAMED_UNIT(*)
SI_UNIT(.CENTI.,.METRE.)
);
#8380=(
NAMED_UNIT(*)
PLANE_ANGLE_UNIT()
SI_UNIT($,.RADIAN.)
);
#8381=(
NAMED_UNIT(*)
SI_UNIT($,.STERADIAN.)
SOLID_ANGLE_UNIT()
);
#8399=SHAPE_DEFINITION_REPRESENTATION(#8430,#8514);
#8430=PRODUCT_DEFINITION_SHAPE('',$,#8546);
#8514=SHAPE_REPRESENTATION('',(#4867),#8363);
#8528=PRODUCT_DEFINITION_CONTEXT('part definition',#8623,'design');
#8546=PRODUCT_DEFINITION('Insert bearing','Insert bearing',#8577,#8528);
#8577=PRODUCT_DEFINITION_FORMATION('',$,#8642);
#8623=APPLICATION_CONTEXT(
'Core Data for Automotive Mechanical Design Process');
#8624=PRODUCT_CONTEXT('part definition',#8623,'mechanical');
#8642=PRODUCT('Insert bearing','Insert bearing','Insert bearing',(#8624));
#8712=COLOUR_RGB('Grey',0.48,0.52,0.57);
#8713=FILL_AREA_STYLE_COLOUR('',#8712);
#8714=FILL_AREA_STYLE('',(#8713));
#8715=SURFACE_STYLE_FILL_AREA(#8714);
#8716=SURFACE_SIDE_STYLE('',(#8715));
#8717=SURFACE_STYLE_USAGE(.BOTH.,#8716);
#8718=PRESENTATION_STYLE_ASSIGNMENT((#8717));
ENDSEC;
END-ISO-10303-21;
